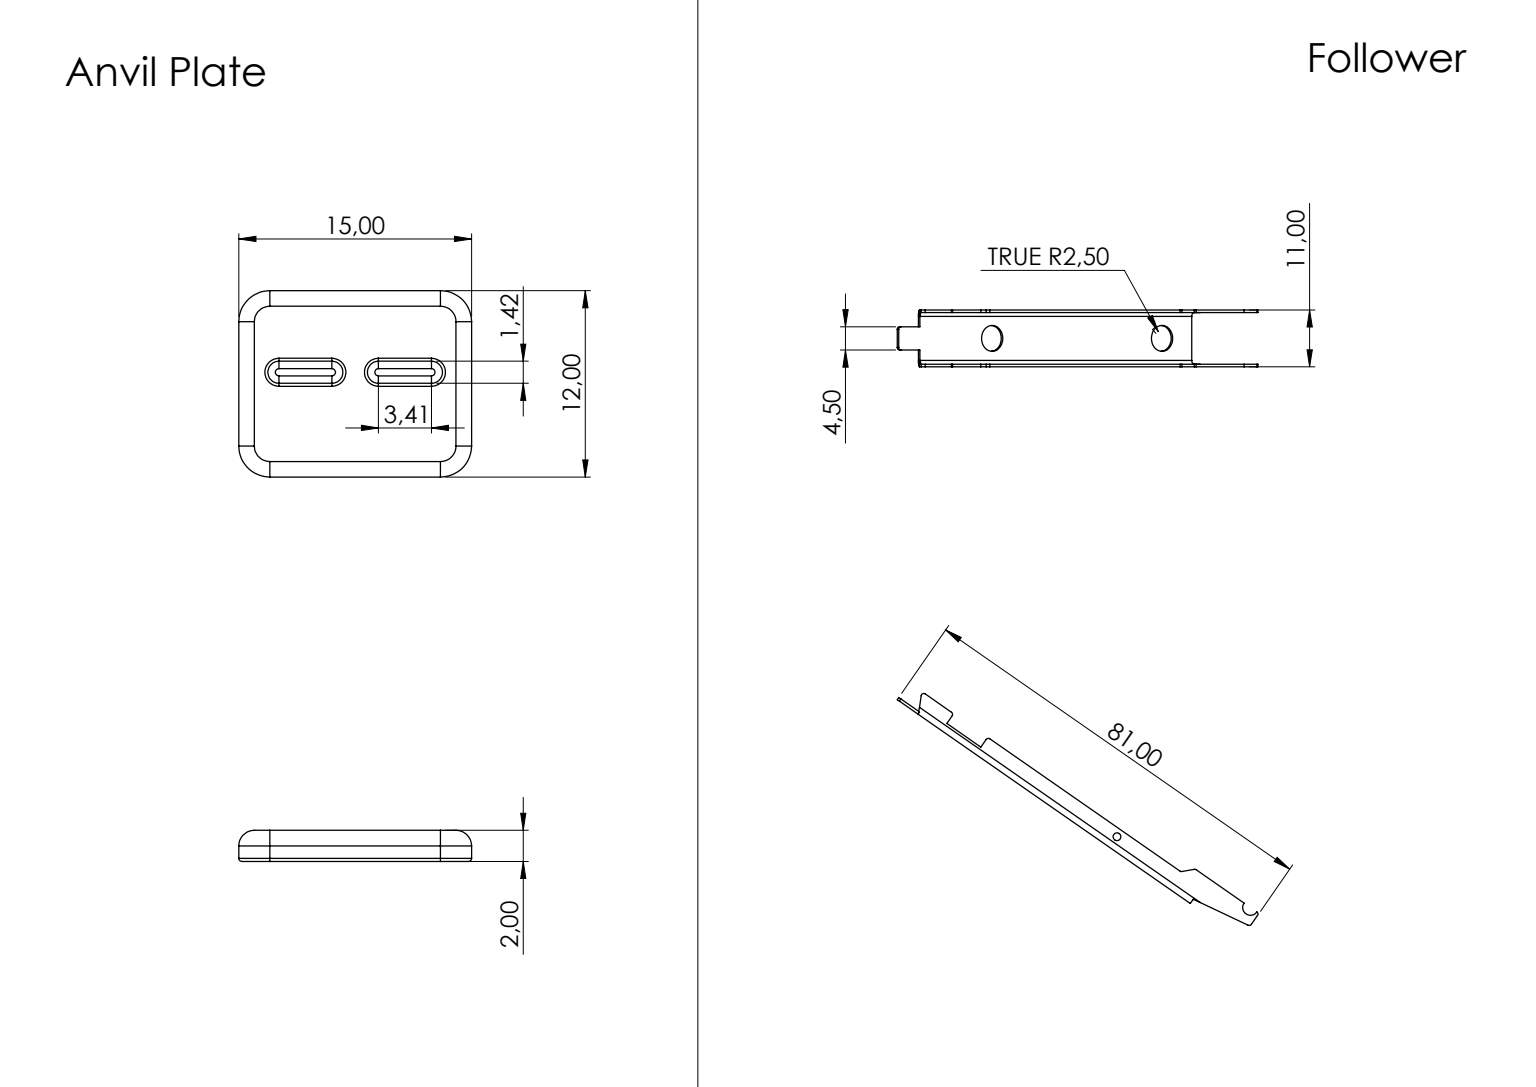
ISO-10303-21;
HEADER;
FILE_DESCRIPTION (('STEP AP214'),
    '1' );
FILE_NAME ('Anvil Plate.step',
    '2026-10-06T10:23:46',
    ( '' ),
    ( '' ),
    'SwSTEP 2.0',
    'SolidWorks 2020',
    '' );
FILE_SCHEMA (( 'AUTOMOTIVE_DESIGN' ));
ENDSEC;

DATA;
#13=EDGE_CURVE ( 'NONE', #2345, #1520, #288, .T. ) ;
#14=DIRECTION ( 'NONE',  ( 0.000000000000000000, 0.000000000000000000, 1.000000000000000000 ) ) ;
#20=CIRCLE ( 'NONE', #15263, 1.000000000000000888 ) ;
#27=CIRCLE ( 'NONE', #15267, 0.2000000000000057288 ) ;
#47=DIRECTION ( 'NONE',  ( 0.000000000000000000, 0.000000000000000000, -1.000000000000000000 ) ) ;
#57=DIRECTION ( 'NONE',  ( 0.000000000000000000, 1.000000000000000000, -3.469446951953613400E-15 ) ) ;
#77=ORIENTED_EDGE ( 'NONE', *, *, #24683, .F. ) ;
#92=ORIENTED_EDGE ( 'NONE', *, *, #24380, .T. ) ;
#97=EDGE_LOOP ( 'NONE', ( #25397, #5551, #19425, #6383 ) ) ;
#102=AXIS2_PLACEMENT_3D ( 'NONE', #15158, #5376, #18644 ) ;
#104=ADVANCED_FACE ( 'NONE', ( #4789 ), #24864, .T. ) ;
#145=CIRCLE ( 'NONE', #6320, 1.000000000000000888 ) ;
#158=AXIS2_PLACEMENT_3D ( 'NONE', #16213, #10429, #24064 ) ;
#165=LINE ( 'NONE', #13580, #21925 ) ;
#168=DIRECTION ( 'NONE',  ( 0.000000000000000000, 1.000000000000000000, -3.469446951953613400E-15 ) ) ;
#183=ORIENTED_EDGE ( 'NONE', *, *, #6628, .F. ) ;
#187=CARTESIAN_POINT ( 'NONE',  ( 43.23147868389327897, 41.90149715599300606, 79.87823623207322044 ) ) ;
#192=DIRECTION ( 'NONE',  ( 0.000000000000000000, 1.000000000000000000, -3.469446951953613400E-15 ) ) ;
#228=CARTESIAN_POINT ( 'NONE',  ( 32.81606138205700773, 36.92314894770294131, 81.17823623207323180 ) ) ;
#229=CYLINDRICAL_SURFACE ( 'NONE', #16961, 0.5000000000000004441 ) ;
#235=VERTEX_POINT ( 'NONE', #24984 ) ;
#237=DIRECTION ( 'NONE',  ( 1.000000000000000000, 0.000000000000000000, 0.000000000000000000 ) ) ;
#251=EDGE_CURVE ( 'NONE', #21293, #8440, #21528, .T. ) ;
#266=AXIS2_PLACEMENT_3D ( 'NONE', #24025, #20423, #700 ) ;
#288=CIRCLE ( 'NONE', #14300, 0.7106531558045068309 ) ;
#305=CARTESIAN_POINT ( 'NONE',  ( -3.469446951953610245E-16, 2.753545109730417678E-13, 79.37823623207336254 ) ) ;
#310=DIRECTION ( 'NONE',  ( 1.000000000000000000, 0.000000000000000000, 0.000000000000000000 ) ) ;
#329=CARTESIAN_POINT ( 'NONE',  ( 31.81606138205700418, 44.92314894770293421, 79.37823623207320622 ) ) ;
#346=EDGE_LOOP ( 'NONE', ( #3037, #6134, #10339, #6691 ) ) ;
#352=CARTESIAN_POINT ( 'NONE',  ( 33.40064408022072939, 41.90149715599300606, 79.37823623207322044 ) ) ;
#373=DIRECTION ( 'NONE',  ( -1.000000000000000000, -0.000000000000000000, -0.000000000000000000 ) ) ;
#407=DIRECTION ( 'NONE',  ( 1.734723475976805122E-16, 3.491481338843134933E-15, 1.000000000000000000 ) ) ;
#425=ADVANCED_FACE ( 'NONE', ( #18305 ), #23824, .T. ) ;
#460=CARTESIAN_POINT ( 'NONE',  ( 36.81465384343994884, 41.67000142393845152, 79.87823623207322044 ) ) ;
#485=TOROIDAL_SURFACE ( 'NONE', #1324, 1.000000000000000000, 1.000000000000000000 ) ;
#492=LINE ( 'NONE', #619, #7832 ) ;
#501=ORIENTED_EDGE ( 'NONE', *, *, #9098, .T. ) ;
#519=CARTESIAN_POINT ( 'NONE',  ( 31.01606138205699992, 44.92314894770294131, 81.17823623207320338 ) ) ;
#544=FACE_OUTER_BOUND ( 'NONE', #14731, .T. ) ;
#551=DIRECTION ( 'NONE',  ( 1.000000000000000000, 0.000000000000000000, 0.000000000000000000 ) ) ;
#565=DIRECTION ( 'NONE',  ( 0.000000000000000000, 0.000000000000000000, 1.000000000000000000 ) ) ;
#590=CARTESIAN_POINT ( 'NONE',  ( 33.40064408022072939, 42.38065457974295924, 79.52109337493035923 ) ) ;
#599=ORIENTED_EDGE ( 'NONE', *, *, #18942, .T. ) ;
#605=EDGE_LOOP ( 'NONE', ( #8949, #22189, #20198, #2594 ) ) ;
#613=CIRCLE ( 'NONE', #19551, 0.2314957320545540931 ) ;
#614=DIRECTION ( 'NONE',  ( 0.000000000000000000, 1.000000000000000000, -3.491481338843134933E-15 ) ) ;
#619=CARTESIAN_POINT ( 'NONE',  ( 43.23147868389327897, 40.76768529863396395, 79.37823623207322044 ) ) ;
#625=EDGE_CURVE ( 'NONE', #9404, #8440, #1536, .T. ) ;
#695=VECTOR ( 'NONE', #8729, 1000.000000000000000 ) ;
#700=DIRECTION ( 'NONE',  ( 0.000000000000000000, 0.000000000000000000, -1.000000000000000000 ) ) ;
#736=DIRECTION ( 'NONE',  ( 0.000000000000000000, 1.000000000000000000, 0.000000000000000000 ) ) ;
#757=DIRECTION ( 'NONE',  ( 0.000000000000000000, 0.000000000000000000, -1.000000000000000000 ) ) ;
#765=CIRCLE ( 'NONE', #17232, 0.5000000000000004441 ) ;
#774=CIRCLE ( 'NONE', #1188, 1.000000000000000888 ) ;
#778=EDGE_LOOP ( 'NONE', ( #24874, #9802, #12952, #15567 ) ) ;
#781=DIRECTION ( 'NONE',  ( 0.000000000000000000, -1.000000000000000000, 0.000000000000000000 ) ) ;
#784=AXIS2_PLACEMENT_3D ( 'NONE', #8790, #6837, #14690 ) ;
#810=ORIENTED_EDGE ( 'NONE', *, *, #4809, .T. ) ;
#822=ORIENTED_EDGE ( 'NONE', *, *, #5627, .F. ) ;
#840=CARTESIAN_POINT ( 'NONE',  ( 43.23147868389327897, 41.90149715599300606, 79.37823623207322044 ) ) ;
#849=CYLINDRICAL_SURFACE ( 'NONE', #21888, 1.000000000000000888 ) ;
#859=DIRECTION ( 'NONE',  ( 0.000000000000000000, -6.938893903907222067E-15, -1.000000000000000000 ) ) ;
#898=EDGE_CURVE ( 'NONE', #1130, #12932, #2769, .T. ) ;
#908=ORIENTED_EDGE ( 'NONE', *, *, #22325, .F. ) ;
#941=EDGE_LOOP ( 'NONE', ( #3944, #19997, #17589, #15115 ) ) ;
#947=VERTEX_POINT ( 'NONE', #19641 ) ;
#961=CARTESIAN_POINT ( 'NONE',  ( 43.81606138205700063, 36.92314894770294131, 81.17823623207323180 ) ) ;
#977=DIRECTION ( 'NONE',  ( 0.000000000000000000, 1.000000000000000000, 0.000000000000000000 ) ) ;
#1014=CARTESIAN_POINT ( 'NONE',  ( 31.81606138205700418, 44.92314894770294131, 80.37823623207322044 ) ) ;
#1056=CARTESIAN_POINT ( 'NONE',  ( 43.23147868389327897, 41.67000142393845152, 79.57823623207323749 ) ) ;
#1057=DIRECTION ( 'NONE',  ( 0.000000000000000000, -3.469446951953613400E-15, -1.000000000000000000 ) ) ;
#1085=VERTEX_POINT ( 'NONE', #2756 ) ;
#1122=CARTESIAN_POINT ( 'NONE',  ( 31.81606138205700418, 36.92314894770294131, 80.37823623207323465 ) ) ;
#1125=DIRECTION ( 'NONE',  ( 0.000000000000000000, 0.000000000000000000, -1.000000000000000000 ) ) ;
#1126=ORIENTED_EDGE ( 'NONE', *, *, #20228, .T. ) ;
#1130=VERTEX_POINT ( 'NONE', #12590 ) ;
#1132=ADVANCED_FACE ( 'NONE', ( #20048 ), #8586, .T. ) ;
#1138=ORIENTED_EDGE ( 'NONE', *, *, #21704, .T. ) ;
#1153=AXIS2_PLACEMENT_3D ( 'NONE', #1229, #14385, #6785 ) ;
#1188=AXIS2_PLACEMENT_3D ( 'NONE', #5142, #18661, #1125 ) ;
#1218=CARTESIAN_POINT ( 'NONE',  ( 33.40064408022072939, 42.57231754924293909, 79.37823623207320622 ) ) ;
#1229=CARTESIAN_POINT ( 'NONE',  ( 32.81606138205700773, 36.92314894770294131, 81.37823623207324886 ) ) ;
#1242=DIRECTION ( 'NONE',  ( 0.000000000000000000, 1.000000000000000000, 0.000000000000000000 ) ) ;
#1280=ORIENTED_EDGE ( 'NONE', *, *, #19495, .T. ) ;
#1323=DIRECTION ( 'NONE',  ( 0.000000000000000000, 0.000000000000000000, 1.000000000000000000 ) ) ;
#1324=AXIS2_PLACEMENT_3D ( 'NONE', #12607, #16567, #16067 ) ;
#1364=ORIENTED_EDGE ( 'NONE', *, *, #18759, .T. ) ;
#1385=EDGE_CURVE ( 'NONE', #23504, #12932, #9806, .T. ) ;
#1393=ORIENTED_EDGE ( 'NONE', *, *, #3030, .T. ) ;
#1416=CARTESIAN_POINT ( 'NONE',  ( 33.40064408022072939, 41.43850569188389699, 79.87823623207322044 ) ) ;
#1474=DIRECTION ( 'NONE',  ( 0.000000000000000000, 0.000000000000000000, -1.000000000000000000 ) ) ;
#1485=ORIENTED_EDGE ( 'NONE', *, *, #2006, .T. ) ;
#1493=DIRECTION ( 'NONE',  ( 1.000000000000000000, 0.000000000000000000, 0.000000000000000000 ) ) ;
#1498=CARTESIAN_POINT ( 'NONE',  ( 32.81606138205700773, 46.92314894770293421, 79.37823623207319201 ) ) ;
#1505=AXIS2_PLACEMENT_3D ( 'NONE', #21822, #6491, #10492 ) ;
#1508=CARTESIAN_POINT ( 'NONE',  ( 45.81606138205700063, 46.92314894770294131, 81.17823623207320338 ) ) ;
#1516=ORIENTED_EDGE ( 'NONE', *, *, #15444, .F. ) ;
#1520=VERTEX_POINT ( 'NONE', #21571 ) ;
#1536=CIRCLE ( 'NONE', #23353, 2.000000000000001776 ) ;
#1587=EDGE_LOOP ( 'NONE', ( #12351, #19325, #9251, #4956 ) ) ;
#1602=AXIS2_PLACEMENT_3D ( 'NONE', #22754, #16570, #1242 ) ;
#1605=EDGE_LOOP ( 'NONE', ( #92, #20381, #12875, #10899 ) ) ;
#1606=ORIENTED_EDGE ( 'NONE', *, *, #898, .F. ) ;
#1608=AXIS2_PLACEMENT_3D ( 'NONE', #10658, #22875, #18507 ) ;
#1612=VERTEX_POINT ( 'NONE', #19892 ) ;
#1669=ADVANCED_FACE ( 'NONE', ( #544 ), #17198, .T. ) ;
#1711=VERTEX_POINT ( 'NONE', #15887 ) ;
#1730=VECTOR ( 'NONE', #2169, 1000.000000000000000 ) ;
#1755=AXIS2_PLACEMENT_3D ( 'NONE', #3524, #11786, #21303 ) ;
#1772=ORIENTED_EDGE ( 'NONE', *, *, #6265, .T. ) ;
#1780=CARTESIAN_POINT ( 'NONE',  ( 36.81465384343994884, 41.67000142393845152, 79.57823623207323749 ) ) ;
#1819=CARTESIAN_POINT ( 'NONE',  ( 43.23147868389327897, 40.76768529863396395, 79.37823623207322044 ) ) ;
#1846=CIRCLE ( 'NONE', #16246, 0.5000000000000004441 ) ;
#1848=VERTEX_POINT ( 'NONE', #17046 ) ;
#1869=DIRECTION ( 'NONE',  ( -0.000000000000000000, -3.469446951953613400E-15, -1.000000000000000000 ) ) ;
#1875=CARTESIAN_POINT ( 'NONE',  ( 43.81606138205700063, 35.92314894770293421, 79.37823623207323465 ) ) ;
#1915=VERTEX_POINT ( 'NONE', #7122 ) ;
#1980=DIRECTION ( 'NONE',  ( 0.000000000000000000, -3.469446951953611033E-15, -1.000000000000000000 ) ) ;
#1984=TOROIDAL_SURFACE ( 'NONE', #17218, 1.000000000000000000, 1.000000000000000000 ) ;
#2000=AXIS2_PLACEMENT_3D ( 'NONE', #9286, #12766, #22537 ) ;
#2006=EDGE_CURVE ( 'NONE', #1520, #12430, #4412, .T. ) ;
#2033=ORIENTED_EDGE ( 'NONE', *, *, #9098, .F. ) ;
#2040=DIRECTION ( 'NONE',  ( 0.000000000000000000, 1.000000000000000000, -3.469446951953613400E-15 ) ) ;
#2042=DIRECTION ( 'NONE',  ( 0.000000000000000000, 3.469446951953613400E-15, 1.000000000000000000 ) ) ;
#2049=ORIENTED_EDGE ( 'NONE', *, *, #4239, .T. ) ;
#2067=DIRECTION ( 'NONE',  ( -0.000000000000000000, -3.469446951953613400E-15, -1.000000000000000000 ) ) ;
#2078=ADVANCED_FACE ( 'NONE', ( #15477 ), #9448, .T. ) ;
#2094=DIRECTION ( 'NONE',  ( 0.000000000000000000, 0.000000000000000000, -1.000000000000000000 ) ) ;
#2121=ORIENTED_EDGE ( 'NONE', *, *, #3983, .T. ) ;
#2142=VECTOR ( 'NONE', #25060, 1000.000000000000000 ) ;
#2154=EDGE_CURVE ( 'NONE', #3400, #23482, #8135, .T. ) ;
#2169=DIRECTION ( 'NONE',  ( -8.758115402030106693E-47, 1.000000000000000000, -3.469446951953613400E-15 ) ) ;
#2176=ORIENTED_EDGE ( 'NONE', *, *, #11481, .F. ) ;
#2182=AXIS2_PLACEMENT_3D ( 'NONE', #14350, #551, #47 ) ;
#2192=CARTESIAN_POINT ( 'NONE',  ( 33.40064408022072939, 42.57231754924293909, 79.37823623207320622 ) ) ;
#2201=AXIS2_PLACEMENT_3D ( 'NONE', #24335, #14817, #6707 ) ;
#2235=PRODUCT_DEFINITION_FORMATION_WITH_SPECIFIED_SOURCE ( 'ANY', '', #3964, .NOT_KNOWN. ) ;
#2249=EDGE_LOOP ( 'NONE', ( #3554, #6520, #9600, #21223 ) ) ;
#2279=CARTESIAN_POINT ( 'NONE',  ( 36.81465384343994884, 42.57231754924293909, 79.57823623207322328 ) ) ;
#2296=DIRECTION ( 'NONE',  ( 1.000000000000000000, -0.000000000000000000, -0.000000000000000000 ) ) ;
#2345=VERTEX_POINT ( 'NONE', #16392 ) ;
#2362=FACE_OUTER_BOUND ( 'NONE', #8970, .T. ) ;
#2364=FACE_OUTER_BOUND ( 'NONE', #2249, .T. ) ;
#2372=EDGE_CURVE ( 'NONE', #24574, #9515, #15507, .T. ) ;
#2380=DIRECTION ( 'NONE',  ( -8.758115402030106693E-47, 1.000000000000000000, -3.469446951953613400E-15 ) ) ;
#2454=CIRCLE ( 'NONE', #11126, 1.800000000000002931 ) ;
#2476=CARTESIAN_POINT ( 'NONE',  ( 32.81606138205700773, 45.92314894770293421, 79.37823623207320622 ) ) ;
#2480=ADVANCED_FACE ( 'NONE', ( #8934 ), #25385, .F. ) ;
#2497=LINE ( 'NONE', #6759, #16866 ) ;
#2528=FACE_OUTER_BOUND ( 'NONE', #778, .T. ) ;
#2533=CIRCLE ( 'NONE', #21472, 0.2000000000000057288 ) ;
#2553=AXIS2_PLACEMENT_3D ( 'NONE', #228, #14278, #21886 ) ;
#2594=ORIENTED_EDGE ( 'NONE', *, *, #5792, .F. ) ;
#2599=CIRCLE ( 'NONE', #7965, 0.2000000000000057288 ) ;
#2614=ADVANCED_FACE ( 'NONE', ( #12934 ), #22453, .F. ) ;
#2671=CARTESIAN_POINT ( 'NONE',  ( 32.81606138205700773, 36.92314894770293421, 79.37823623207323465 ) ) ;
#2691=DIRECTION ( 'NONE',  ( 0.000000000000000000, 0.000000000000000000, -1.000000000000000000 ) ) ;
#2725=DIRECTION ( 'NONE',  ( 0.000000000000000000, 1.000000000000000000, -3.469446951953613400E-15 ) ) ;
#2756=CARTESIAN_POINT ( 'NONE',  ( 30.81606138205700418, 44.92314894770294131, 80.37823623207322044 ) ) ;
#2757=VERTEX_POINT ( 'NONE', #15227 ) ;
#2763=ORIENTED_EDGE ( 'NONE', *, *, #11568, .F. ) ;
#2766=DIRECTION ( 'NONE',  ( 0.000000000000000000, 1.000000000000000000, -3.469446951953613400E-15 ) ) ;
#2769=LINE ( 'NONE', #16829, #695 ) ;
#2811=DIRECTION ( 'NONE',  ( 0.000000000000000000, 0.000000000000000000, 1.000000000000000000 ) ) ;
#2854=ORIENTED_EDGE ( 'NONE', *, *, #24360, .T. ) ;
#2907=ORIENTED_EDGE ( 'NONE', *, *, #20730, .T. ) ;
#2913=VECTOR ( 'NONE', #10280, 1000.000000000000000 ) ;
#2941=ORIENTED_EDGE ( 'NONE', *, *, #898, .T. ) ;
#2983=AXIS2_PLACEMENT_3D ( 'NONE', #20163, #8189, #565 ) ;
#3008=DIRECTION ( 'NONE',  ( 0.000000000000000000, 0.000000000000000000, 1.000000000000000000 ) ) ;
#3029=DIRECTION ( 'NONE',  ( 0.000000000000000000, -3.469446951953613400E-15, -1.000000000000000000 ) ) ;
#3030=EDGE_CURVE ( 'NONE', #7575, #19237, #18812, .T. ) ;
#3036=ORIENTED_EDGE ( 'NONE', *, *, #5474, .F. ) ;
#3037=ORIENTED_EDGE ( 'NONE', *, *, #7448, .F. ) ;
#3049=AXIS2_PLACEMENT_3D ( 'NONE', #8952, #9089, #8704 ) ;
#3069=UNCERTAINTY_MEASURE_WITH_UNIT (LENGTH_MEASURE( 1.000000000000000082E-05 ), #19515, 'distance_accuracy_value', 'NONE');
#3073=EDGE_CURVE ( 'NONE', #6274, #19237, #5359, .T. ) ;
#3285=DIRECTION ( 'NONE',  ( 0.000000000000000000, 1.000000000000000000, 0.000000000000000000 ) ) ;
#3301=DIRECTION ( 'NONE',  ( 0.000000000000000000, 1.000000000000000000, 0.000000000000000000 ) ) ;
#3315=DIRECTION ( 'NONE',  ( -0.000000000000000000, -3.469446951953613400E-15, -1.000000000000000000 ) ) ;
#3345=CIRCLE ( 'NONE', #19383, 0.5000000000000004441 ) ;
#3354=CARTESIAN_POINT ( 'NONE',  ( 39.81746892067405952, 42.57231754924293909, 79.37823623207320622 ) ) ;
#3387=VECTOR ( 'NONE', #13615, 1000.000000000000000 ) ;
#3394=CIRCLE ( 'NONE', #21099, 0.2000000000000057288 ) ;
#3400=VERTEX_POINT ( 'NONE', #5923 ) ;
#3404=( NAMED_UNIT ( * ) SI_UNIT ( $, .STERADIAN. ) SOLID_ANGLE_UNIT ( ) );
#3439=CARTESIAN_POINT ( 'NONE',  ( 36.81465384343994884, 40.76768529863396395, 79.37823623207322044 ) ) ;
#3473=PLANE ( 'NONE',  #18226 ) ;
#3482=ORIENTED_EDGE ( 'NONE', *, *, #13193, .T. ) ;
#3503=DIRECTION ( 'NONE',  ( -1.000000000000000000, 0.000000000000000000, 0.000000000000000000 ) ) ;
#3524=CARTESIAN_POINT ( 'NONE',  ( 39.81746892067405952, 42.57231754924293909, 79.57823623207322328 ) ) ;
#3534=DIRECTION ( 'NONE',  ( 0.000000000000000000, -1.000000000000000000, 0.000000000000000000 ) ) ;
#3537=( NAMED_UNIT ( * ) PLANE_ANGLE_UNIT ( ) SI_UNIT ( $, .RADIAN. ) );
#3554=ORIENTED_EDGE ( 'NONE', *, *, #13651, .T. ) ;
#3567=EDGE_CURVE ( 'NONE', #11430, #8412, #21363, .T. ) ;
#3569=AXIS2_PLACEMENT_3D ( 'NONE', #6497, #7937, #4190 ) ;
#3614=DIRECTION ( 'NONE',  ( 0.000000000000000000, 1.000000000000000000, 0.000000000000000000 ) ) ;
#3622=ORIENTED_EDGE ( 'NONE', *, *, #14918, .T. ) ;
#3690=ORIENTED_EDGE ( 'NONE', *, *, #17616, .T. ) ;
#3691=ORIENTED_EDGE ( 'NONE', *, *, #12095, .F. ) ;
#3692=CARTESIAN_POINT ( 'NONE',  ( 36.81465384343994884, 40.76768529863396395, 79.37823623207322044 ) ) ;
#3777=FILL_AREA_STYLE_COLOUR ( '', #11896 ) ;
#3785=VERTEX_POINT ( 'NONE', #10145 ) ;
#3800=CIRCLE ( 'NONE', #16984, 1.000000000000000888 ) ;
#3835=VERTEX_POINT ( 'NONE', #5541 ) ;
#3849=EDGE_LOOP ( 'NONE', ( #1772, #15717, #7269, #22855 ) ) ;
#3883=CIRCLE ( 'NONE', #18291, 1.000000000000000888 ) ;
#3890=DIRECTION ( 'NONE',  ( 0.000000000000000000, 0.000000000000000000, 1.000000000000000000 ) ) ;
#3896=LINE ( 'NONE', #23842, #15599 ) ;
#3922=ADVANCED_FACE ( 'NONE', ( #21372 ), #23415, .T. ) ;
#3944=ORIENTED_EDGE ( 'NONE', *, *, #16305, .T. ) ;
#3959=DIRECTION ( 'NONE',  ( 1.000000000000000000, 0.000000000000000000, 0.000000000000000000 ) ) ;
#3963=FACE_OUTER_BOUND ( 'NONE', #11280, .T. ) ;
#3964=PRODUCT ( 'Anvil Plate', 'Anvil Plate', '', ( #21040 ) ) ;
#3983=EDGE_CURVE ( 'NONE', #947, #1085, #19708, .T. ) ;
#4075=CARTESIAN_POINT ( 'NONE',  ( 39.81746892067405952, 41.67000142393845152, 79.57823623207323749 ) ) ;
#4097=FACE_OUTER_BOUND ( 'NONE', #18488, .T. ) ;
#4143=EDGE_CURVE ( 'NONE', #24976, #13846, #18108, .T. ) ;
#4190=DIRECTION ( 'NONE',  ( 0.000000000000000000, 1.000000000000000000, -3.469446951953613400E-15 ) ) ;
#4212=EDGE_LOOP ( 'NONE', ( #15416, #8055, #7794, #2176 ) ) ;
#4234=CIRCLE ( 'NONE', #14102, 1.000000000000000888 ) ;
#4239=EDGE_CURVE ( 'NONE', #9789, #15078, #2497, .T. ) ;
#4260=ORIENTED_EDGE ( 'NONE', *, *, #5474, .T. ) ;
#4277=CARTESIAN_POINT ( 'NONE',  ( 39.81746892067405952, 42.57231754924293909, 79.37823623207320622 ) ) ;
#4302=ORIENTED_EDGE ( 'NONE', *, *, #7371, .F. ) ;
#4355=CARTESIAN_POINT ( 'NONE',  ( 43.23147868389327897, 40.95934826813394380, 79.52109337493037344 ) ) ;
#4368=FACE_OUTER_BOUND ( 'NONE', #1587, .T. ) ;
#4412=CIRCLE ( 'NONE', #19209, 0.2000000000000057288 ) ;
#4450=CYLINDRICAL_SURFACE ( 'NONE', #5529, 0.2000000000000057288 ) ;
#4480=CARTESIAN_POINT ( 'NONE',  ( 39.81746892067405952, 40.76768529863396395, 79.37823623207322044 ) ) ;
#4496=FACE_OUTER_BOUND ( 'NONE', #6721, .T. ) ;
#4499=CARTESIAN_POINT ( 'NONE',  ( 45.61606138205700489, 44.92314894770294131, 81.17823623207320338 ) ) ;
#4527=LINE ( 'NONE', #18185, #7625 ) ;
#4539=VECTOR ( 'NONE', #14558, 1000.000000000000000 ) ;
#4566=EDGE_CURVE ( 'NONE', #1711, #21638, #19744, .T. ) ;
#4578=PLANE ( 'NONE',  #7457 ) ;
#4613=AXIS2_PLACEMENT_3D ( 'NONE', #5567, #2067, #9570 ) ;
#4672=DIRECTION ( 'NONE',  ( 0.000000000000000000, 0.000000000000000000, -1.000000000000000000 ) ) ;
#4693=CIRCLE ( 'NONE', #15330, 0.2000000000000057288 ) ;
#4699=ORIENTED_EDGE ( 'NONE', *, *, #4143, .F. ) ;
#4705=DIRECTION ( 'NONE',  ( -1.000000000000000000, 0.000000000000000000, 0.000000000000000000 ) ) ;
#4739=LINE ( 'NONE', #12612, #5832 ) ;
#4747=CARTESIAN_POINT ( 'NONE',  ( 45.81606138205700063, 34.92314894770293421, 79.37823623207323465 ) ) ;
#4762=DIRECTION ( 'NONE',  ( 1.000000000000000000, -0.000000000000000000, 0.000000000000000000 ) ) ;
#4787=CARTESIAN_POINT ( 'NONE',  ( 39.81746892067405952, 41.67000142393845152, 79.37823623207322044 ) ) ;
#4789=FACE_OUTER_BOUND ( 'NONE', #346, .T. ) ;
#4801=DIRECTION ( 'NONE',  ( 1.000000000000000000, 0.000000000000000000, -0.000000000000000000 ) ) ;
#4806=VECTOR ( 'NONE', #10198, 1000.000000000000000 ) ;
#4809=EDGE_CURVE ( 'NONE', #12932, #5707, #19729, .T. ) ;
#4879=EDGE_LOOP ( 'NONE', ( #20930, #20768, #17898, #4699 ) ) ;
#4882=CIRCLE ( 'NONE', #19283, 0.2314957320545540931 ) ;
#4932=VECTOR ( 'NONE', #17827, 1000.000000000000000 ) ;
#4956=ORIENTED_EDGE ( 'NONE', *, *, #18759, .F. ) ;
#4968=DIRECTION ( 'NONE',  ( 0.000000000000000000, 1.000000000000000000, -3.469446951953613400E-15 ) ) ;
#4974=CIRCLE ( 'NONE', #25113, 1.000000000000000888 ) ;
#4986=ADVANCED_FACE ( 'NONE', ( #14831 ), #20892, .F. ) ;
#4998=DIRECTION ( 'NONE',  ( 0.000000000000000000, 1.000000000000000000, 0.000000000000000000 ) ) ;
#5000=DIRECTION ( 'NONE',  ( 0.000000000000000000, -1.000000000000000000, 6.938893903907221278E-15 ) ) ;
#5026=CARTESIAN_POINT ( 'NONE',  ( 43.23147868389327897, 42.57231754924293909, 79.57823623207325170 ) ) ;
#5028=DIRECTION ( 'NONE',  ( -1.000000000000000000, 0.000000000000000000, 0.000000000000000000 ) ) ;
#5118=DIRECTION ( 'NONE',  ( 1.000000000000000000, 0.000000000000000000, 0.000000000000000000 ) ) ;
#5142=CARTESIAN_POINT ( 'NONE',  ( 43.81606138205700063, 35.92314894770294131, 80.37823623207323465 ) ) ;
#5143=VERTEX_POINT ( 'NONE', #7623 ) ;
#5146=EDGE_LOOP ( 'NONE', ( #23125, #7873, #11574, #23348 ) ) ;
#5175=ORIENTED_EDGE ( 'NONE', *, *, #5481, .F. ) ;
#5222=EDGE_LOOP ( 'NONE', ( #1126, #12846, #10725, #7105 ) ) ;
#5288=CIRCLE ( 'NONE', #1153, 1.800000000000002931 ) ;
#5359=CIRCLE ( 'NONE', #7767, 1.000000000000000888 ) ;
#5374=ORIENTED_EDGE ( 'NONE', *, *, #14624, .T. ) ;
#5376=DIRECTION ( 'NONE',  ( -0.000000000000000000, -3.469446951953613400E-15, -1.000000000000000000 ) ) ;
#5382=DIRECTION ( 'NONE',  ( 1.000000000000000000, -0.000000000000000000, -0.000000000000000000 ) ) ;
#5385=LINE ( 'NONE', #1498, #2142 ) ;
#5395=ORIENTED_EDGE ( 'NONE', *, *, #15441, .F. ) ;
#5424=EDGE_CURVE ( 'NONE', #13993, #1915, #14022, .T. ) ;
#5435=VECTOR ( 'NONE', #6960, 1000.000000000000000 ) ;
#5449=DIRECTION ( 'NONE',  ( -1.000000000000000000, 0.000000000000000000, 0.000000000000000000 ) ) ;
#5457=VECTOR ( 'NONE', #24680, 1000.000000000000000 ) ;
#5474=EDGE_CURVE ( 'NONE', #1520, #5143, #23469, .T. ) ;
#5481=EDGE_CURVE ( 'NONE', #19237, #8412, #20, .T. ) ;
#5482=FILL_AREA_STYLE ('',( #19256 ) ) ;
#5523=COLOUR_RGB ( '', 0.08235294, 0.09019608, 0.10196078) ;
#5529=AXIS2_PLACEMENT_3D ( 'NONE', #10249, #4705, #12317 ) ;
#5541=CARTESIAN_POINT ( 'NONE',  ( 32.81606138205700773, 46.92314894770294131, 81.17823623207318917 ) ) ;
#5551=ORIENTED_EDGE ( 'NONE', *, *, #24334, .F. ) ;
#5567=CARTESIAN_POINT ( 'NONE',  ( 43.81606138205700063, 44.92314894770294131, 81.17823623207320338 ) ) ;
#5570=CARTESIAN_POINT ( 'NONE',  ( 43.23147868389327897, 40.76768529863396395, 79.57823623207325170 ) ) ;
#5573=ADVANCED_FACE ( 'NONE', ( #15662 ), #17739, .T. ) ;
#5597=PRODUCT_DEFINITION_SHAPE ( 'NONE', 'NONE',  #23001 ) ;
#5599=EDGE_LOOP ( 'NONE', ( #1485, #22225, #16839, #23920 ) ) ;
#5627=EDGE_CURVE ( 'NONE', #6274, #24574, #17868, .T. ) ;
#5653=VECTOR ( 'NONE', #21399, 1000.000000000000000 ) ;
#5707=VERTEX_POINT ( 'NONE', #19918 ) ;
#5730=SHAPE_REPRESENTATION_RELATIONSHIP ( 'NONE' , 'NONE' ,  #10983, #9253 ) ;
#5792=EDGE_CURVE ( 'NONE', #1915, #16335, #8452, .T. ) ;
#5805=CARTESIAN_POINT ( 'NONE',  ( 33.40064408022072939, 40.95934826813394380, 79.52109337493035923 ) ) ;
#5821=DIRECTION ( 'NONE',  ( 0.000000000000000000, 1.000000000000000000, 0.000000000000000000 ) ) ;
#5832=VECTOR ( 'NONE', #20451, 1000.000000000000000 ) ;
#5865=LINE ( 'NONE', #20023, #9019 ) ;
#5890=ORIENTED_EDGE ( 'NONE', *, *, #5424, .T. ) ;
#5897=DIRECTION ( 'NONE',  ( 1.000000000000000000, -0.000000000000000000, 0.000000000000000000 ) ) ;
#5903=TOROIDAL_SURFACE ( 'NONE', #17027, 0.9023161253044896801, 0.2000000000000000111 ) ;
#5923=CARTESIAN_POINT ( 'NONE',  ( 43.23147868389327897, 42.57231754924293909, 79.37823623207320622 ) ) ;
#5965=CARTESIAN_POINT ( 'NONE',  ( 44.81606138205700063, 36.92314894770293421, 79.37823623207323465 ) ) ;
#5966=ADVANCED_FACE ( 'NONE', ( #15122 ), #12826, .T. ) ;
#5995=DIRECTION ( 'NONE',  ( 8.758115402030106693E-47, -1.000000000000000000, 3.469446951953613400E-15 ) ) ;
#6068=CARTESIAN_POINT ( 'NONE',  ( -3.469446951953610245E-16, 45.92314894770294131, 80.37823623207322044 ) ) ;
#6086=EDGE_CURVE ( 'NONE', #22567, #10123, #22398, .T. ) ;
#6134=ORIENTED_EDGE ( 'NONE', *, *, #9957, .F. ) ;
#6207=CIRCLE ( 'NONE', #21427, 1.000000000000000888 ) ;
#6242=DIRECTION ( 'NONE',  ( 1.000000000000000000, 0.000000000000000000, -0.000000000000000000 ) ) ;
#6248=FACE_BOUND ( 'NONE', #12703, .T. ) ;
#6250=EDGE_LOOP ( 'NONE', ( #15505, #9557, #24312, #22938 ) ) ;
#6261=VECTOR ( 'NONE', #20515, 1000.000000000000000 ) ;
#6263=AXIS2_PLACEMENT_3D ( 'NONE', #4787, #20508, #25073 ) ;
#6265=EDGE_CURVE ( 'NONE', #11430, #1915, #6362, .T. ) ;
#6266=LINE ( 'NONE', #24481, #6261 ) ;
#6272=EDGE_CURVE ( 'NONE', #22152, #17202, #3883, .T. ) ;
#6274=VERTEX_POINT ( 'NONE', #6731 ) ;
#6286=CIRCLE ( 'NONE', #7950, 0.2000000000000057288 ) ;
#6294=TOROIDAL_SURFACE ( 'NONE', #2553, 1.800000000000000044, 0.2000000000000000111 ) ;
#6315=CARTESIAN_POINT ( 'NONE',  ( 45.81606138205700063, 36.92314894770294131, 81.17823623207321759 ) ) ;
#6320=AXIS2_PLACEMENT_3D ( 'NONE', #1014, #20863, #12891 ) ;
#6336=CIRCLE ( 'NONE', #2201, 2.000000000000001776 ) ;
#6362=LINE ( 'NONE', #14335, #11719 ) ;
#6383=ORIENTED_EDGE ( 'NONE', *, *, #13, .F. ) ;
#6386=FACE_OUTER_BOUND ( 'NONE', #10307, .T. ) ;
#6419=DIRECTION ( 'NONE',  ( -1.000000000000000000, 0.000000000000000000, -0.000000000000000000 ) ) ;
#6467=CARTESIAN_POINT ( 'NONE',  ( 33.40064408022072939, 41.67000142393845152, 79.37823623207322044 ) ) ;
#6468=TOROIDAL_SURFACE ( 'NONE', #9357, 0.2314957320545545372, 0.5000000000000000000 ) ;
#6491=DIRECTION ( 'NONE',  ( 0.000000000000000000, 3.469446951953613400E-15, 1.000000000000000000 ) ) ;
#6497=CARTESIAN_POINT ( 'NONE',  ( 43.81606138205700063, 44.92314894770294131, 81.17823623207320338 ) ) ;
#6520=ORIENTED_EDGE ( 'NONE', *, *, #7973, .F. ) ;
#6531=CARTESIAN_POINT ( 'NONE',  ( 43.23147868389327897, 41.67000142393845152, 79.37823623207322044 ) ) ;
#6534=FACE_OUTER_BOUND ( 'NONE', #13113, .T. ) ;
#6562=AXIS2_PLACEMENT_3D ( 'NONE', #10788, #12984, #977 ) ;
#6602=DIRECTION ( 'NONE',  ( 0.000000000000000000, 1.000000000000000000, 0.000000000000000000 ) ) ;
#6603=DIRECTION ( 'NONE',  ( 1.734723475976805122E-16, 3.491481338843134933E-15, 1.000000000000000000 ) ) ;
#6628=EDGE_CURVE ( 'NONE', #13616, #5143, #613, .T. ) ;
#6678=ORIENTED_EDGE ( 'NONE', *, *, #3073, .F. ) ;
#6691=ORIENTED_EDGE ( 'NONE', *, *, #8106, .F. ) ;
#6707=DIRECTION ( 'NONE',  ( 0.000000000000000000, 1.000000000000000000, 0.000000000000000000 ) ) ;
#6721=EDGE_LOOP ( 'NONE', ( #11827, #21729, #21136, #13228 ) ) ;
#6731=CARTESIAN_POINT ( 'NONE',  ( 32.81606138205700773, 34.92314894770294131, 80.37823623207323465 ) ) ;
#6759=CARTESIAN_POINT ( 'NONE',  ( 0.000000000000000000, 35.12314894770293705, 81.37823623207324886 ) ) ;
#6785=DIRECTION ( 'NONE',  ( 0.000000000000000000, 1.000000000000000000, 0.000000000000000000 ) ) ;
#6786=EDGE_CURVE ( 'NONE', #13846, #10306, #15970, .T. ) ;
#6792=CARTESIAN_POINT ( 'NONE',  ( 32.81606138205700773, 44.92314894770294131, 81.37823623207322044 ) ) ;
#6798=FACE_OUTER_BOUND ( 'NONE', #11554, .T. ) ;
#6804=CARTESIAN_POINT ( 'NONE',  ( 32.81606138205700773, 35.12314894770294416, 81.37823623207324886 ) ) ;
#6833=CARTESIAN_POINT ( 'NONE',  ( 32.81606138205700773, 35.92314894770293421, 79.37823623207323465 ) ) ;
#6837=DIRECTION ( 'NONE',  ( 0.000000000000000000, 3.469446951953613400E-15, 1.000000000000000000 ) ) ;
#6867=EDGE_CURVE ( 'NONE', #1130, #19369, #1846, .T. ) ;
#6937=( GEOMETRIC_REPRESENTATION_CONTEXT ( 3 ) GLOBAL_UNCERTAINTY_ASSIGNED_CONTEXT ( ( #18240 ) ) GLOBAL_UNIT_ASSIGNED_CONTEXT ( ( #19502, #17076, #3404 ) ) REPRESENTATION_CONTEXT ( 'NONE', 'WORKASPACE' ) );
#6945=AXIS2_PLACEMENT_3D ( 'NONE', #24755, #5449, #1323 ) ;
#6947=DIRECTION ( 'NONE',  ( -0.000000000000000000, -3.469446951953613400E-15, -1.000000000000000000 ) ) ;
#6955=FACE_OUTER_BOUND ( 'NONE', #10604, .T. ) ;
#6960=DIRECTION ( 'NONE',  ( 8.758115402030106693E-47, -1.000000000000000000, 3.469446951953613400E-15 ) ) ;
#7000=DIRECTION ( 'NONE',  ( -8.758115402030106693E-47, 1.000000000000000000, -3.469446951953613400E-15 ) ) ;
#7022=CARTESIAN_POINT ( 'NONE',  ( 33.40064408022072939, 41.43850569188389699, 79.37823623207322044 ) ) ;
#7038=CARTESIAN_POINT ( 'NONE',  ( 39.81746892067405952, 42.38065457974295924, 79.52109337493037344 ) ) ;
#7058=CARTESIAN_POINT ( 'NONE',  ( 43.81606138205700063, 36.92314894770293421, 79.37823623207323465 ) ) ;
#7074=DIRECTION ( 'NONE',  ( 0.000000000000000000, 1.000000000000000000, 0.000000000000000000 ) ) ;
#7105=ORIENTED_EDGE ( 'NONE', *, *, #23720, .T. ) ;
#7111=ORIENTED_EDGE ( 'NONE', *, *, #16308, .T. ) ;
#7122=CARTESIAN_POINT ( 'NONE',  ( 30.81606138205700418, 36.92314894770294131, 81.17823623207323180 ) ) ;
#7143=FACE_OUTER_BOUND ( 'NONE', #23302, .T. ) ;
#7174=FACE_OUTER_BOUND ( 'NONE', #15055, .T. ) ;
#7269=ORIENTED_EDGE ( 'NONE', *, *, #14948, .T. ) ;
#7295=ORIENTED_EDGE ( 'NONE', *, *, #11580, .T. ) ;
#7339=EDGE_LOOP ( 'NONE', ( #24898, #24455, #14377, #24400 ) ) ;
#7344=AXIS2_PLACEMENT_3D ( 'NONE', #21061, #7533, #21188 ) ;
#7365=CARTESIAN_POINT ( 'NONE',  ( 43.81606138205700063, 46.92314894770293421, 79.37823623207319201 ) ) ;
#7371=EDGE_CURVE ( 'NONE', #1612, #13993, #20713, .T. ) ;
#7448=EDGE_CURVE ( 'NONE', #24976, #19369, #3394, .T. ) ;
#7451=ORIENTED_EDGE ( 'NONE', *, *, #11713, .F. ) ;
#7457=AXIS2_PLACEMENT_3D ( 'NONE', #305, #20289, #57 ) ;
#7494=AXIS2_PLACEMENT_3D ( 'NONE', #6792, #24671, #3301 ) ;
#7501=ORIENTED_EDGE ( 'NONE', *, *, #6272, .T. ) ;
#7504=SHAPE_DEFINITION_REPRESENTATION ( #5597, #10983 ) ;
#7530=DIRECTION ( 'NONE',  ( 1.000000000000000000, 0.000000000000000000, 0.000000000000000000 ) ) ;
#7533=DIRECTION ( 'NONE',  ( 1.000000000000000000, 0.000000000000000000, 0.000000000000000000 ) ) ;
#7575=VERTEX_POINT ( 'NONE', #1875 ) ;
#7592=AXIS2_PLACEMENT_3D ( 'NONE', #9094, #9224, #3008 ) ;
#7623=CARTESIAN_POINT ( 'NONE',  ( 43.23147868389327897, 41.43850569188389699, 79.87823623207322044 ) ) ;
#7625=VECTOR ( 'NONE', #8653, 1000.000000000000000 ) ;
#7670=SURFACE_STYLE_FILL_AREA ( #5482 ) ;
#7717=LINE ( 'NONE', #9909, #12848 ) ;
#7737=ORIENTED_EDGE ( 'NONE', *, *, #20228, .F. ) ;
#7743=EDGE_CURVE ( 'NONE', #2757, #13616, #6266, .T. ) ;
#7767=AXIS2_PLACEMENT_3D ( 'NONE', #9168, #10959, #22549 ) ;
#7794=ORIENTED_EDGE ( 'NONE', *, *, #16305, .F. ) ;
#7798=SURFACE_STYLE_USAGE ( .BOTH. , #9484 ) ;
#7832=VECTOR ( 'NONE', #237, 1000.000000000000000 ) ;
#7873=ORIENTED_EDGE ( 'NONE', *, *, #5424, .F. ) ;
#7895=EDGE_CURVE ( 'NONE', #1085, #11430, #15473, .T. ) ;
#7927=CIRCLE ( 'NONE', #7494, 1.800000000000002931 ) ;
#7937=DIRECTION ( 'NONE',  ( -0.000000000000000000, -3.469446951953613400E-15, -1.000000000000000000 ) ) ;
#7943=AXIS2_PLACEMENT_3D ( 'NONE', #460, #23907, #22237 ) ;
#7950=AXIS2_PLACEMENT_3D ( 'NONE', #8453, #23894, #19920 ) ;
#7952=EDGE_LOOP ( 'NONE', ( #13257, #15522, #18354, #1606 ) ) ;
#7965=AXIS2_PLACEMENT_3D ( 'NONE', #14476, #16524, #12567 ) ;
#7968=CARTESIAN_POINT ( 'NONE',  ( 36.81465384343994884, 40.95934826813394380, 79.52109337493037344 ) ) ;
#7973=EDGE_CURVE ( 'NONE', #9136, #3785, #2454, .T. ) ;
#8012=ORIENTED_EDGE ( 'NONE', *, *, #24661, .T. ) ;
#8049=ORIENTED_EDGE ( 'NONE', *, *, #17211, .T. ) ;
#8055=ORIENTED_EDGE ( 'NONE', *, *, #19946, .F. ) ;
#8065=FACE_OUTER_BOUND ( 'NONE', #23914, .T. ) ;
#8075=ORIENTED_EDGE ( 'NONE', *, *, #4143, .T. ) ;
#8082=ORIENTED_EDGE ( 'NONE', *, *, #21225, .T. ) ;
#8094=DIRECTION ( 'NONE',  ( 0.000000000000000000, 1.000000000000000000, 0.000000000000000000 ) ) ;
#8106=EDGE_CURVE ( 'NONE', #19369, #23504, #10194, .T. ) ;
#8135=LINE ( 'NONE', #4277, #4806 ) ;
#8177=AXIS2_PLACEMENT_3D ( 'NONE', #12636, #15761, #21567 ) ;
#8189=DIRECTION ( 'NONE',  ( -1.000000000000000000, 0.000000000000000000, 0.000000000000000000 ) ) ;
#8210=DIRECTION ( 'NONE',  ( -8.758115402030106693E-47, 1.000000000000000000, -3.469446951953613400E-15 ) ) ;
#8220=ORIENTED_EDGE ( 'NONE', *, *, #12827, .T. ) ;
#8246=CARTESIAN_POINT ( 'NONE',  ( 45.81606138205700063, 44.92314894770294131, 81.17823623207320338 ) ) ;
#8250=CIRCLE ( 'NONE', #9925, 0.9023161253044892360 ) ;
#8270=DIRECTION ( 'NONE',  ( -0.000000000000000000, -3.469446951953613400E-15, -1.000000000000000000 ) ) ;
#8308=DIRECTION ( 'NONE',  ( 0.000000000000000000, 0.000000000000000000, -1.000000000000000000 ) ) ;
#8350=LINE ( 'NONE', #4355, #2913 ) ;
#8412=VERTEX_POINT ( 'NONE', #17386 ) ;
#8440=VERTEX_POINT ( 'NONE', #11732 ) ;
#8452=LINE ( 'NONE', #20168, #20595 ) ;
#8453=CARTESIAN_POINT ( 'NONE',  ( 43.81606138205700063, 35.12314894770293705, 81.17823623207323180 ) ) ;
#8475=CARTESIAN_POINT ( 'NONE',  ( 33.40064408022072939, 40.76768529863396395, 79.37823623207322044 ) ) ;
#8483=DIRECTION ( 'NONE',  ( -0.000000000000000000, -3.469446951953613400E-15, -1.000000000000000000 ) ) ;
#8516=DIRECTION ( 'NONE',  ( 0.000000000000000000, 1.000000000000000000, -3.469446951953613400E-15 ) ) ;
#8561=DIRECTION ( 'NONE',  ( 0.000000000000000000, 0.000000000000000000, 1.000000000000000000 ) ) ;
#8586=CYLINDRICAL_SURFACE ( 'NONE', #266, 0.2000000000000057288 ) ;
#8635=AXIS2_PLACEMENT_3D ( 'NONE', #14455, #17955, #781 ) ;
#8653=DIRECTION ( 'NONE',  ( 1.000000000000000000, 0.000000000000000000, 0.000000000000000000 ) ) ;
#8704=DIRECTION ( 'NONE',  ( 1.734723475976805122E-16, 0.000000000000000000, 1.000000000000000000 ) ) ;
#8729=DIRECTION ( 'NONE',  ( -1.000000000000000000, 0.000000000000000000, 0.000000000000000000 ) ) ;
#8734=DIRECTION ( 'NONE',  ( 0.000000000000000000, 1.000000000000000000, -3.469446951953613400E-15 ) ) ;
#8740=DIRECTION ( 'NONE',  ( 0.000000000000000000, 3.469446951953611033E-15, 1.000000000000000000 ) ) ;
#8782=DIRECTION ( 'NONE',  ( -1.000000000000000000, 0.000000000000000000, 0.000000000000000000 ) ) ;
#8785=CIRCLE ( 'NONE', #21120, 0.2000000000000057288 ) ;
#8790=CARTESIAN_POINT ( 'NONE',  ( 33.40064408022072939, 41.67000142393845152, 79.37823623207322044 ) ) ;
#8819=DIRECTION ( 'NONE',  ( 0.000000000000000000, 0.000000000000000000, -1.000000000000000000 ) ) ;
#8934=FACE_OUTER_BOUND ( 'NONE', #11469, .T. ) ;
#8949=ORIENTED_EDGE ( 'NONE', *, *, #10543, .F. ) ;
#8952=CARTESIAN_POINT ( 'NONE',  ( 45.81606138205700063, 46.92314894770293421, 79.37823623207319201 ) ) ;
#8970=EDGE_LOOP ( 'NONE', ( #7111, #17634, #22349, #9503 ) ) ;
#8971=CARTESIAN_POINT ( 'NONE',  ( 31.01606138205700347, 44.92314894770294131, 81.37823623207322044 ) ) ;
#9019=VECTOR ( 'NONE', #13724, 1000.000000000000000 ) ;
#9026=CARTESIAN_POINT ( 'NONE',  ( 36.81465384343994884, 41.43850569188389699, 79.37823623207322044 ) ) ;
#9049=ORIENTED_EDGE ( 'NONE', *, *, #16308, .F. ) ;
#9061=DIRECTION ( 'NONE',  ( 1.000000000000000000, 0.000000000000000000, -0.000000000000000000 ) ) ;
#9078=CYLINDRICAL_SURFACE ( 'NONE', #25208, 0.2000000000000057288 ) ;
#9089=DIRECTION ( 'NONE',  ( -1.000000000000000000, 6.018531076210103283E-31, 1.734723475976805122E-16 ) ) ;
#9094=CARTESIAN_POINT ( 'NONE',  ( 43.23147868389327897, 40.76768529863396395, 79.57823623207323749 ) ) ;
#9098=EDGE_CURVE ( 'NONE', #24470, #2345, #4527, .T. ) ;
#9125=VERTEX_POINT ( 'NONE', #16482 ) ;
#9136=VERTEX_POINT ( 'NONE', #20234 ) ;
#9163=DIRECTION ( 'NONE',  ( -0.000000000000000000, -3.469446951953613400E-15, -1.000000000000000000 ) ) ;
#9168=CARTESIAN_POINT ( 'NONE',  ( 32.81606138205700773, 35.92314894770294131, 80.37823623207323465 ) ) ;
#9170=DIRECTION ( 'NONE',  ( 1.734723475976805122E-16, 3.491481338843134933E-15, 1.000000000000000000 ) ) ;
#9186=CARTESIAN_POINT ( 'NONE',  ( 30.81606138205700418, 46.92314894770293421, 79.37823623207319201 ) ) ;
#9224=DIRECTION ( 'NONE',  ( -1.000000000000000000, 0.000000000000000000, 0.000000000000000000 ) ) ;
#9251=ORIENTED_EDGE ( 'NONE', *, *, #9367, .F. ) ;
#9253=ADVANCED_BREP_SHAPE_REPRESENTATION ( '', ( #25350, #2000 ), #16613 ) ;
#9286=CARTESIAN_POINT ( 'NONE',  ( 0.000000000000000000, 0.000000000000000000, 0.000000000000000000 ) ) ;
#9357=AXIS2_PLACEMENT_3D ( 'NONE', #6467, #18446, #16756 ) ;
#9367=EDGE_CURVE ( 'NONE', #235, #12986, #13280, .T. ) ;
#9388=AXIS2_PLACEMENT_3D ( 'NONE', #16011, #17967, #168 ) ;
#9404=VERTEX_POINT ( 'NONE', #22801 ) ;
#9448=PLANE ( 'NONE',  #17158 ) ;
#9484=SURFACE_SIDE_STYLE ('',( #7670 ) ) ;
#9503=ORIENTED_EDGE ( 'NONE', *, *, #7895, .F. ) ;
#9515=VERTEX_POINT ( 'NONE', #21503 ) ;
#9519=CARTESIAN_POINT ( 'NONE',  ( 43.81606138205700063, 45.92314894770293421, 79.37823623207320622 ) ) ;
#9552=ADVANCED_FACE ( 'NONE', ( #13779 ), #3473, .F. ) ;
#9557=ORIENTED_EDGE ( 'NONE', *, *, #14726, .F. ) ;
#9570=DIRECTION ( 'NONE',  ( 0.000000000000000000, 1.000000000000000000, 0.000000000000000000 ) ) ;
#9598=ADVANCED_FACE ( 'NONE', ( #18155 ), #6294, .T. ) ;
#9600=ORIENTED_EDGE ( 'NONE', *, *, #13243, .F. ) ;
#9604=CIRCLE ( 'NONE', #158, 0.2000000000000057288 ) ;
#9670=ORIENTED_EDGE ( 'NONE', *, *, #3073, .T. ) ;
#9678=DIRECTION ( 'NONE',  ( 0.000000000000000000, 0.000000000000000000, 1.000000000000000000 ) ) ;
#9712=ORIENTED_EDGE ( 'NONE', *, *, #20420, .F. ) ;
#9729=CARTESIAN_POINT ( 'NONE',  ( 31.01606138205699992, 36.92314894770294131, 81.17823623207323180 ) ) ;
#9789=VERTEX_POINT ( 'NONE', #6804 ) ;
#9802=ORIENTED_EDGE ( 'NONE', *, *, #20730, .F. ) ;
#9806=CIRCLE ( 'NONE', #22534, 0.5000000000000004441 ) ;
#9820=DIRECTION ( 'NONE',  ( 8.758115402030106693E-47, -1.000000000000000000, 3.469446951953613400E-15 ) ) ;
#9857=EDGE_CURVE ( 'NONE', #21638, #7575, #4234, .T. ) ;
#9866=CARTESIAN_POINT ( 'NONE',  ( 43.81606138205700063, 46.92314894770294131, 81.17823623207318917 ) ) ;
#9880=ORIENTED_EDGE ( 'NONE', *, *, #14297, .T. ) ;
#9908=EDGE_LOOP ( 'NONE', ( #9880, #15629, #23440, #15210 ) ) ;
#9909=CARTESIAN_POINT ( 'NONE',  ( 45.81606138205700063, 44.92314894770293421, 79.37823623207320622 ) ) ;
#9925=AXIS2_PLACEMENT_3D ( 'NONE', #6531, #14390, #8094 ) ;
#9957=EDGE_CURVE ( 'NONE', #17769, #24976, #23523, .T. ) ;
#9995=FACE_OUTER_BOUND ( 'NONE', #19170, .T. ) ;
#10007=CARTESIAN_POINT ( 'NONE',  ( 30.81606138205700418, 44.92314894770293421, 79.37823623207320622 ) ) ;
#10032=ORIENTED_EDGE ( 'NONE', *, *, #3567, .T. ) ;
#10110=VERTEX_POINT ( 'NONE', #10267 ) ;
#10120=ORIENTED_EDGE ( 'NONE', *, *, #25442, .F. ) ;
#10123=VERTEX_POINT ( 'NONE', #13876 ) ;
#10145=CARTESIAN_POINT ( 'NONE',  ( 43.81606138205700063, 46.72314894770294558, 81.37823623207320622 ) ) ;
#10194=LINE ( 'NONE', #24327, #4539 ) ;
#10198=DIRECTION ( 'NONE',  ( -1.000000000000000000, 0.000000000000000000, 0.000000000000000000 ) ) ;
#10211=LINE ( 'NONE', #23972, #11839 ) ;
#10222=CYLINDRICAL_SURFACE ( 'NONE', #15768, 2.000000000000001776 ) ;
#10249=CARTESIAN_POINT ( 'NONE',  ( 45.81606138205700063, 35.12314894770293705, 81.17823623207323180 ) ) ;
#10256=FACE_OUTER_BOUND ( 'NONE', #10786, .T. ) ;
#10267=CARTESIAN_POINT ( 'NONE',  ( 39.81746892067405952, 41.43850569188389699, 79.87823623207322044 ) ) ;
#10270=CARTESIAN_POINT ( 'NONE',  ( 31.01606138205699992, 36.92314894770294131, 81.37823623207324886 ) ) ;
#10271=AXIS2_PLACEMENT_3D ( 'NONE', #1122, #5000, #859 ) ;
#10280=DIRECTION ( 'NONE',  ( -1.000000000000000000, 0.000000000000000000, 0.000000000000000000 ) ) ;
#10282=VERTEX_POINT ( 'NONE', #8971 ) ;
#10302=ORIENTED_EDGE ( 'NONE', *, *, #3983, .F. ) ;
#10306=VERTEX_POINT ( 'NONE', #1218 ) ;
#10307=EDGE_LOOP ( 'NONE', ( #8049, #4302, #18356, #18215 ) ) ;
#10339=ORIENTED_EDGE ( 'NONE', *, *, #13272, .F. ) ;
#10357=CYLINDRICAL_SURFACE ( 'NONE', #2182, 0.2000000000000057288 ) ;
#10388=TOROIDAL_SURFACE ( 'NONE', #11624, 0.9023161253044896801, 0.2000000000000000111 ) ;
#10398=LINE ( 'NONE', #329, #20293 ) ;
#10421=ADVANCED_FACE ( 'NONE', ( #20556 ), #23559, .T. ) ;
#10429=DIRECTION ( 'NONE',  ( -1.000000000000000000, 0.000000000000000000, 0.000000000000000000 ) ) ;
#10452=DIRECTION ( 'NONE',  ( -0.000000000000000000, -3.469446951953613400E-15, -1.000000000000000000 ) ) ;
#10457=VECTOR ( 'NONE', #9170, 1000.000000000000000 ) ;
#10483=LINE ( 'NONE', #14462, #12072 ) ;
#10492=DIRECTION ( 'NONE',  ( 0.000000000000000000, 1.000000000000000000, 0.000000000000000000 ) ) ;
#10543=EDGE_CURVE ( 'NONE', #11605, #1915, #14144, .T. ) ;
#10548=DIRECTION ( 'NONE',  ( 0.000000000000000000, 0.000000000000000000, -1.000000000000000000 ) ) ;
#10561=ORIENTED_EDGE ( 'NONE', *, *, #15581, .F. ) ;
#10593=AXIS2_PLACEMENT_3D ( 'NONE', #16520, #1057, #16658 ) ;
#10604=EDGE_LOOP ( 'NONE', ( #9670, #21631, #908, #822 ) ) ;
#10606=CARTESIAN_POINT ( 'NONE',  ( 32.81606138205700773, 44.92314894770293421, 79.37823623207320622 ) ) ;
#10658=CARTESIAN_POINT ( 'NONE',  ( 33.40064408022072939, 41.67000142393845152, 79.87823623207322044 ) ) ;
#10706=CARTESIAN_POINT ( 'NONE',  ( 43.81606138205700063, 45.92314894770293421, 80.37823623207322044 ) ) ;
#10710=FACE_OUTER_BOUND ( 'NONE', #1605, .T. ) ;
#10725=ORIENTED_EDGE ( 'NONE', *, *, #6628, .T. ) ;
#10727=ORIENTED_EDGE ( 'NONE', *, *, #13193, .F. ) ;
#10757=ADVANCED_FACE ( 'NONE', ( #24613 ), #5903, .T. ) ;
#10786=EDGE_LOOP ( 'NONE', ( #15532, #8220, #22506, #25370 ) ) ;
#10788=CARTESIAN_POINT ( 'NONE',  ( 36.81465384343994884, 41.67000142393845152, 79.37823623207322044 ) ) ;
#10870=ORIENTED_EDGE ( 'NONE', *, *, #11241, .F. ) ;
#10884=PLANE ( 'NONE',  #3049 ) ;
#10899=ORIENTED_EDGE ( 'NONE', *, *, #9857, .F. ) ;
#10959=DIRECTION ( 'NONE',  ( 1.000000000000000000, 0.000000000000000000, 0.000000000000000000 ) ) ;
#10983=SHAPE_REPRESENTATION ( 'Anvil Plate', ( #2000 ), #16613 ) ;
#11036=AXIS2_PLACEMENT_3D ( 'NONE', #16857, #8270, #13125 ) ;
#11051=ORIENTED_EDGE ( 'NONE', *, *, #12598, .T. ) ;
#11055=ADVANCED_FACE ( 'NONE', ( #13653 ), #15792, .F. ) ;
#11101=ADVANCED_FACE ( 'NONE', ( #4368 ), #229, .F. ) ;
#11107=DIRECTION ( 'NONE',  ( 1.000000000000000000, -6.018531076210103283E-31, -1.734723475976805122E-16 ) ) ;
#11126=AXIS2_PLACEMENT_3D ( 'NONE', #21404, #15857, #5821 ) ;
#11155=ADVANCED_FACE ( 'NONE', ( #4496 ), #15952, .F. ) ;
#11220=AXIS2_PLACEMENT_3D ( 'NONE', #2279, #6419, #18385 ) ;
#11223=AXIS2_PLACEMENT_3D ( 'NONE', #13149, #5028, #16746 ) ;
#11232=CIRCLE ( 'NONE', #15743, 2.000000000000001776 ) ;
#11241=EDGE_CURVE ( 'NONE', #9515, #9404, #22394, .T. ) ;
#11280=EDGE_LOOP ( 'NONE', ( #11783, #24766, #4260, #183 ) ) ;
#11282=CIRCLE ( 'NONE', #14955, 1.000000000000000888 ) ;
#11298=PRESENTATION_STYLE_ASSIGNMENT (( #7798 ) ) ;
#11413=( LENGTH_UNIT ( ) NAMED_UNIT ( * ) SI_UNIT ( .MILLI., .METRE. ) );
#11424=CLOSED_SHELL ( 'NONE', ( #4986, #22630, #13704, #11155, #24727, #9552, #18224, #15165, #15608, #17115, #17498, #425, #23172, #19469, #17813, #14745, #16321, #17628, #22832, #2078, #11101, #11055, #21857, #2614, #13633, #2480, #19481, #24415, #104, #17772, #3922, #20278, #12739, #10757, #5573, #5966, #12318, #1669, #9598, #12264, #13606, #21360, #10421, #1132 ) ) ;
#11430=VERTEX_POINT ( 'NONE', #14655 ) ;
#11448=VECTOR ( 'NONE', #24150, 1000.000000000000000 ) ;
#11469=EDGE_LOOP ( 'NONE', ( #22198, #18960, #10727, #7737 ) ) ;
#11472=DIRECTION ( 'NONE',  ( 0.000000000000000000, -3.469446951953613400E-15, -1.000000000000000000 ) ) ;
#11481=EDGE_CURVE ( 'NONE', #17202, #1848, #17500, .T. ) ;
#11506=DIRECTION ( 'NONE',  ( 0.000000000000000000, 1.000000000000000000, -3.469446951953613400E-15 ) ) ;
#11554=EDGE_LOOP ( 'NONE', ( #8012, #10870, #12642, #23769 ) ) ;
#11555=CARTESIAN_POINT ( 'NONE',  ( 44.81606138205700063, 44.92314894770293421, 80.37823623207322044 ) ) ;
#11568=EDGE_CURVE ( 'NONE', #17202, #947, #3800, .T. ) ;
#11570=AXIS2_PLACEMENT_3D ( 'NONE', #4075, #1869, #192 ) ;
#11574=ORIENTED_EDGE ( 'NONE', *, *, #17211, .F. ) ;
#11580=EDGE_CURVE ( 'NONE', #947, #3835, #5385, .T. ) ;
#11602=CARTESIAN_POINT ( 'NONE',  ( 36.81465384343994884, 42.38065457974295924, 79.52109337493035923 ) ) ;
#11605=VERTEX_POINT ( 'NONE', #10270 ) ;
#11624=AXIS2_PLACEMENT_3D ( 'NONE', #24290, #18273, #8734 ) ;
#11646=EDGE_CURVE ( 'NONE', #8412, #22152, #10398, .T. ) ;
#11694=VERTEX_POINT ( 'NONE', #590 ) ;
#11713=EDGE_CURVE ( 'NONE', #235, #1130, #12887, .T. ) ;
#11719=VECTOR ( 'NONE', #407, 1000.000000000000000 ) ;
#11732=CARTESIAN_POINT ( 'NONE',  ( 43.81606138205700063, 46.92314894770294131, 80.37823623207322044 ) ) ;
#11783=ORIENTED_EDGE ( 'NONE', *, *, #15398, .F. ) ;
#11786=DIRECTION ( 'NONE',  ( -1.000000000000000000, 0.000000000000000000, -0.000000000000000000 ) ) ;
#11799=CARTESIAN_POINT ( 'NONE',  ( 32.81606138205700773, 44.92314894770294131, 81.17823623207320338 ) ) ;
#11809=ORIENTED_EDGE ( 'NONE', *, *, #19821, .F. ) ;
#11816=DIRECTION ( 'NONE',  ( 1.000000000000000000, -0.000000000000000000, -0.000000000000000000 ) ) ;
#11827=ORIENTED_EDGE ( 'NONE', *, *, #12974, .T. ) ;
#11839=VECTOR ( 'NONE', #19606, 1000.000000000000000 ) ;
#11842=ORIENTED_EDGE ( 'NONE', *, *, #9957, .T. ) ;
#11861=CARTESIAN_POINT ( 'NONE',  ( 36.81465384343994884, 41.67000142393845152, 79.37823623207322044 ) ) ;
#11896=COLOUR_RGB ( '', 0.08235294, 0.09019608, 0.10196078) ;
#11958=ORIENTED_EDGE ( 'NONE', *, *, #18218, .T. ) ;
#11994=CARTESIAN_POINT ( 'NONE',  ( 39.81746892067405952, 41.90149715599300606, 79.37823623207322044 ) ) ;
#12072=VECTOR ( 'NONE', #22318, 1000.000000000000000 ) ;
#12095=EDGE_CURVE ( 'NONE', #16335, #3835, #11232, .T. ) ;
#12121=AXIS2_PLACEMENT_3D ( 'NONE', #18115, #310, #23887 ) ;
#12264=ADVANCED_FACE ( 'NONE', ( #24116 ), #10357, .T. ) ;
#12317=DIRECTION ( 'NONE',  ( 0.000000000000000000, 0.000000000000000000, 1.000000000000000000 ) ) ;
#12318=ADVANCED_FACE ( 'NONE', ( #12686 ), #9078, .T. ) ;
#12351=ORIENTED_EDGE ( 'NONE', *, *, #24955, .F. ) ;
#12368=DIRECTION ( 'NONE',  ( 0.000000000000000000, 3.491481338843134933E-15, 1.000000000000000000 ) ) ;
#12405=EDGE_CURVE ( 'NONE', #3835, #19999, #2599, .T. ) ;
#12430=VERTEX_POINT ( 'NONE', #1819 ) ;
#12486=AXIS2_PLACEMENT_3D ( 'NONE', #961, #24522, #4968 ) ;
#12530=AXIS2_PLACEMENT_3D ( 'NONE', #11994, #20082, #9678 ) ;
#12567=DIRECTION ( 'NONE',  ( 0.000000000000000000, 0.000000000000000000, -1.000000000000000000 ) ) ;
#12586=CARTESIAN_POINT ( 'NONE',  ( 43.81606138205700063, 36.92314894770293421, 79.37823623207322044 ) ) ;
#12590=CARTESIAN_POINT ( 'NONE',  ( 36.81465384343994884, 41.43850569188389699, 79.87823623207322044 ) ) ;
#12598=EDGE_CURVE ( 'NONE', #16335, #10282, #8785, .T. ) ;
#12607=CARTESIAN_POINT ( 'NONE',  ( 32.81606138205700773, 36.92314894770294131, 80.37823623207323465 ) ) ;
#12612=CARTESIAN_POINT ( 'NONE',  ( 45.81606138205700063, 36.92314894770293421, 79.37823623207323465 ) ) ;
#12636=CARTESIAN_POINT ( 'NONE',  ( 32.81606138205700773, 36.92314894770294131, 80.37823623207323465 ) ) ;
#12642=ORIENTED_EDGE ( 'NONE', *, *, #24380, .F. ) ;
#12652=CARTESIAN_POINT ( 'NONE',  ( 43.23147868389327897, 42.57231754924293909, 79.57823623207323749 ) ) ;
#12686=FACE_OUTER_BOUND ( 'NONE', #605, .T. ) ;
#12703=EDGE_LOOP ( 'NONE', ( #8075, #22847, #2907, #11842 ) ) ;
#12710=MECHANICAL_DESIGN_GEOMETRIC_PRESENTATION_REPRESENTATION('',(#22987),#6937);
#12723=DIRECTION ( 'NONE',  ( 1.000000000000000000, 6.938893903907222067E-15, 0.000000000000000000 ) ) ;
#12739=ADVANCED_FACE ( 'NONE', ( #24088 ), #20491, .T. ) ;
#12763=CARTESIAN_POINT ( 'NONE',  ( 32.81606138205700773, 36.92314894770293421, 79.37823623207323465 ) ) ;
#12764=AXIS2_PLACEMENT_3D ( 'NONE', #23754, #5995, #1980 ) ;
#12766=DIRECTION ( 'NONE',  ( 0.000000000000000000, 0.000000000000000000, 1.000000000000000000 ) ) ;
#12826=CYLINDRICAL_SURFACE ( 'NONE', #7592, 0.2000000000000057288 ) ;
#12827=EDGE_CURVE ( 'NONE', #23772, #1612, #6336, .T. ) ;
#12846=ORIENTED_EDGE ( 'NONE', *, *, #7743, .T. ) ;
#12848=VECTOR ( 'NONE', #23541, 1000.000000000000000 ) ;
#12864=DIRECTION ( 'NONE',  ( 1.734723475976805122E-16, 3.491481338843134933E-15, 1.000000000000000000 ) ) ;
#12875=ORIENTED_EDGE ( 'NONE', *, *, #22325, .T. ) ;
#12880=ORIENTED_EDGE ( 'NONE', *, *, #15581, .T. ) ;
#12887=CIRCLE ( 'NONE', #7943, 0.2314957320545540931 ) ;
#12891=DIRECTION ( 'NONE',  ( 0.000000000000000000, -6.938893903907222067E-15, -1.000000000000000000 ) ) ;
#12892=AXIS2_PLACEMENT_3D ( 'NONE', #23227, #7530, #2094 ) ;
#12896=DIRECTION ( 'NONE',  ( 0.000000000000000000, 1.000000000000000000, -3.469446951953613400E-15 ) ) ;
#12902=DIRECTION ( 'NONE',  ( 0.000000000000000000, 0.000000000000000000, -1.000000000000000000 ) ) ;
#12920=DIRECTION ( 'NONE',  ( 0.000000000000000000, 1.000000000000000000, 0.000000000000000000 ) ) ;
#12932=VERTEX_POINT ( 'NONE', #1416 ) ;
#12934=FACE_OUTER_BOUND ( 'NONE', #7952, .T. ) ;
#12952=ORIENTED_EDGE ( 'NONE', *, *, #25366, .F. ) ;
#12970=CARTESIAN_POINT ( 'NONE',  ( 36.81465384343994884, 41.90149715599300606, 79.87823623207322044 ) ) ;
#12974=EDGE_CURVE ( 'NONE', #24574, #1612, #17140, .T. ) ;
#12984=DIRECTION ( 'NONE',  ( 0.000000000000000000, 3.469446951953613400E-15, 1.000000000000000000 ) ) ;
#12986=VERTEX_POINT ( 'NONE', #11602 ) ;
#12996=CARTESIAN_POINT ( 'NONE',  ( 43.81606138205700063, 36.92314894770294131, 81.37823623207324886 ) ) ;
#13027=ORIENTED_EDGE ( 'NONE', *, *, #17919, .T. ) ;
#13113=EDGE_LOOP ( 'NONE', ( #10032, #5175, #6678, #10120 ) ) ;
#13115=DIRECTION ( 'NONE',  ( 0.000000000000000000, 0.000000000000000000, -1.000000000000000000 ) ) ;
#13125=DIRECTION ( 'NONE',  ( 0.000000000000000000, 1.000000000000000000, 0.000000000000000000 ) ) ;
#13149=CARTESIAN_POINT ( 'NONE',  ( 36.81465384343994884, 41.90149715599300606, 79.37823623207322044 ) ) ;
#13177=VECTOR ( 'NONE', #8782, 1000.000000000000000 ) ;
#13193=EDGE_CURVE ( 'NONE', #2757, #24470, #17040, .T. ) ;
#13227=AXIS2_PLACEMENT_3D ( 'NONE', #840, #5118, #14517 ) ;
#13228=ORIENTED_EDGE ( 'NONE', *, *, #5627, .T. ) ;
#13240=ORIENTED_EDGE ( 'NONE', *, *, #12405, .F. ) ;
#13243=EDGE_CURVE ( 'NONE', #23789, #9136, #4693, .T. ) ;
#13257=ORIENTED_EDGE ( 'NONE', *, *, #6867, .T. ) ;
#13271=VECTOR ( 'NONE', #3959, 1000.000000000000000 ) ;
#13272=EDGE_CURVE ( 'NONE', #23504, #17769, #9604, .T. ) ;
#13275=DIRECTION ( 'NONE',  ( -0.000000000000000000, -3.469446951953613400E-15, -1.000000000000000000 ) ) ;
#13280=CIRCLE ( 'NONE', #11223, 0.5000000000000004441 ) ;
#13330=CARTESIAN_POINT ( 'NONE',  ( 36.81465384343994884, 42.57231754924293909, 79.37823623207320622 ) ) ;
#13335=AXIS2_PLACEMENT_3D ( 'NONE', #16475, #18428, #757 ) ;
#13351=( NAMED_UNIT ( * ) SI_UNIT ( $, .STERADIAN. ) SOLID_ANGLE_UNIT ( ) );
#13355=AXIS2_PLACEMENT_3D ( 'NONE', #20390, #16009, #24230 ) ;
#13358=EDGE_LOOP ( 'NONE', ( #14739, #2941, #810, #1364 ) ) ;
#13465=( NAMED_UNIT ( * ) SI_UNIT ( $, .STERADIAN. ) SOLID_ANGLE_UNIT ( ) );
#13500=CARTESIAN_POINT ( 'NONE',  ( 32.81606138205700773, 35.92314894770293421, 79.37823623207323465 ) ) ;
#13525=CIRCLE ( 'NONE', #7344, 0.2000000000000057288 ) ;
#13580=CARTESIAN_POINT ( 'NONE',  ( 45.61606138205700489, 2.823374736507280597E-13, 81.37823623207336254 ) ) ;
#13606=ADVANCED_FACE ( 'NONE', ( #6386 ), #4450, .T. ) ;
#13607=DIRECTION ( 'NONE',  ( 6.938893903907221278E-15, -1.000000000000000000, 0.000000000000000000 ) ) ;
#13615=DIRECTION ( 'NONE',  ( -1.734723475976805122E-16, -3.491481338843134933E-15, -1.000000000000000000 ) ) ;
#13616=VERTEX_POINT ( 'NONE', #187 ) ;
#13633=ADVANCED_FACE ( 'NONE', ( #8065 ), #17983, .F. ) ;
#13651=EDGE_CURVE ( 'NONE', #21293, #3785, #17398, .T. ) ;
#13653=FACE_OUTER_BOUND ( 'NONE', #17452, .T. ) ;
#13704=ADVANCED_FACE ( 'NONE', ( #7143 ), #10884, .F. ) ;
#13724=DIRECTION ( 'NONE',  ( -1.000000000000000000, -0.000000000000000000, 0.000000000000000000 ) ) ;
#13759=DIRECTION ( 'NONE',  ( 0.000000000000000000, 0.000000000000000000, -1.000000000000000000 ) ) ;
#13779=FACE_OUTER_BOUND ( 'NONE', #14962, .T. ) ;
#13798=ORIENTED_EDGE ( 'NONE', *, *, #9367, .T. ) ;
#13846=VERTEX_POINT ( 'NONE', #13330 ) ;
#13876=CARTESIAN_POINT ( 'NONE',  ( 39.81746892067405952, 40.95934826813394380, 79.52109337493035923 ) ) ;
#13955=EDGE_LOOP ( 'NONE', ( #13987, #5395, #24658, #23942 ) ) ;
#13957=FACE_OUTER_BOUND ( 'NONE', #23760, .T. ) ;
#13987=ORIENTED_EDGE ( 'NONE', *, *, #13243, .T. ) ;
#13993=VERTEX_POINT ( 'NONE', #23475 ) ;
#14004=ORIENTED_EDGE ( 'NONE', *, *, #17764, .T. ) ;
#14022=CIRCLE ( 'NONE', #15668, 2.000000000000001776 ) ;
#14061=CIRCLE ( 'NONE', #4613, 2.000000000000001776 ) ;
#14075=AXIS2_PLACEMENT_3D ( 'NONE', #14811, #9163, #12896 ) ;
#14102=AXIS2_PLACEMENT_3D ( 'NONE', #7058, #3315, #736 ) ;
#14144=CIRCLE ( 'NONE', #21129, 0.2000000000000057288 ) ;
#14192=CARTESIAN_POINT ( 'NONE',  ( 32.81606138205700773, 44.92314894770294131, 80.37823623207322044 ) ) ;
#14249=DIRECTION ( 'NONE',  ( 1.734723475976805122E-16, 3.491481338843134933E-15, 1.000000000000000000 ) ) ;
#14278=DIRECTION ( 'NONE',  ( -0.000000000000000000, -3.469446951953613400E-15, -1.000000000000000000 ) ) ;
#14288=LINE ( 'NONE', #16086, #15186 ) ;
#14297=EDGE_CURVE ( 'NONE', #23482, #22567, #15701, .T. ) ;
#14300=AXIS2_PLACEMENT_3D ( 'NONE', #16507, #15089, #12920 ) ;
#14303=AXIS2_PLACEMENT_3D ( 'NONE', #2671, #12864, #24687 ) ;
#14335=CARTESIAN_POINT ( 'NONE',  ( 30.81606138205700418, 36.92314894770293421, 79.37823623207323465 ) ) ;
#14350=CARTESIAN_POINT ( 'NONE',  ( 45.81606138205700063, 46.72314894770294558, 81.17823623207318917 ) ) ;
#14377=ORIENTED_EDGE ( 'NONE', *, *, #24955, .T. ) ;
#14385=DIRECTION ( 'NONE',  ( 0.000000000000000000, 3.469446951953613400E-15, 1.000000000000000000 ) ) ;
#14386=EDGE_CURVE ( 'NONE', #9404, #23789, #7717, .T. ) ;
#14390=DIRECTION ( 'NONE',  ( 0.000000000000000000, 3.469446951953613400E-15, 1.000000000000000000 ) ) ;
#14455=CARTESIAN_POINT ( 'NONE',  ( 33.40064408022072939, 41.67000142393845152, 79.87823623207322044 ) ) ;
#14462=CARTESIAN_POINT ( 'NONE',  ( 0.000000000000000000, 46.72314894770294558, 81.37823623207320622 ) ) ;
#14476=CARTESIAN_POINT ( 'NONE',  ( 32.81606138205700773, 46.72314894770294558, 81.17823623207320338 ) ) ;
#14486=ORIENTED_EDGE ( 'NONE', *, *, #7973, .T. ) ;
#14503=ORIENTED_EDGE ( 'NONE', *, *, #7743, .F. ) ;
#14517=DIRECTION ( 'NONE',  ( 0.000000000000000000, 0.000000000000000000, -1.000000000000000000 ) ) ;
#14549=DIRECTION ( 'NONE',  ( -0.000000000000000000, -3.469446951953613400E-15, -1.000000000000000000 ) ) ;
#14554=CYLINDRICAL_SURFACE ( 'NONE', #13335, 1.000000000000000888 ) ;
#14558=DIRECTION ( 'NONE',  ( -1.000000000000000000, -0.000000000000000000, 0.000000000000000000 ) ) ;
#14624=EDGE_CURVE ( 'NONE', #23772, #9515, #4739, .T. ) ;
#14647=CARTESIAN_POINT ( 'NONE',  ( 39.81746892067405952, 41.67000142393845152, 79.52109337493035923 ) ) ;
#14655=CARTESIAN_POINT ( 'NONE',  ( 30.81606138205700418, 36.92314894770294131, 80.37823623207322044 ) ) ;
#14664=UNCERTAINTY_MEASURE_WITH_UNIT (LENGTH_MEASURE( 1.000000000000000082E-05 ), #11413, 'distance_accuracy_value', 'NONE');
#14690=DIRECTION ( 'NONE',  ( 0.000000000000000000, 1.000000000000000000, 0.000000000000000000 ) ) ;
#14726=EDGE_CURVE ( 'NONE', #10123, #24470, #15299, .T. ) ;
#14731=EDGE_LOOP ( 'NONE', ( #11051, #21985, #13240, #3691 ) ) ;
#14739=ORIENTED_EDGE ( 'NONE', *, *, #11713, .T. ) ;
#14745=ADVANCED_FACE ( 'NONE', ( #6798 ), #849, .T. ) ;
#14795=LINE ( 'NONE', #1508, #24652 ) ;
#14811=CARTESIAN_POINT ( 'NONE',  ( 43.81606138205700063, 36.92314894770294131, 80.37823623207323465 ) ) ;
#14817=DIRECTION ( 'NONE',  ( -0.000000000000000000, -3.469446951953613400E-15, -1.000000000000000000 ) ) ;
#14831=FACE_OUTER_BOUND ( 'NONE', #3849, .T. ) ;
#14871=DIRECTION ( 'NONE',  ( 0.000000000000000000, 0.000000000000000000, 1.000000000000000000 ) ) ;
#14903=CARTESIAN_POINT ( 'NONE',  ( 36.81465384343994884, 40.76768529863396395, 79.57823623207323749 ) ) ;
#14918=EDGE_CURVE ( 'NONE', #12986, #19369, #23553, .T. ) ;
#14942=DIRECTION ( 'NONE',  ( 1.000000000000000000, 0.000000000000000000, 0.000000000000000000 ) ) ;
#14948=EDGE_CURVE ( 'NONE', #16335, #1085, #15913, .T. ) ;
#14955=AXIS2_PLACEMENT_3D ( 'NONE', #10706, #4762, #2691 ) ;
#14962=EDGE_LOOP ( 'NONE', ( #11958, #16123, #14486, #12880, #13027, #3690, #1280, #2049 ) ) ;
#15055=EDGE_LOOP ( 'NONE', ( #3482, #501, #20157, #14503 ) ) ;
#15078=VERTEX_POINT ( 'NONE', #18122 ) ;
#15089=DIRECTION ( 'NONE',  ( -0.000000000000000000, -3.469446951953613400E-15, -1.000000000000000000 ) ) ;
#15115=ORIENTED_EDGE ( 'NONE', *, *, #18942, .F. ) ;
#15122=FACE_OUTER_BOUND ( 'NONE', #5599, .T. ) ;
#15133=ORIENTED_EDGE ( 'NONE', *, *, #4566, .T. ) ;
#15151=EDGE_CURVE ( 'NONE', #15078, #1612, #6286, .T. ) ;
#15158=CARTESIAN_POINT ( 'NONE',  ( 36.81465384343994884, 41.67000142393845152, 79.52109337493035923 ) ) ;
#15165=ADVANCED_FACE ( 'NONE', ( #10256 ), #18366, .T. ) ;
#15186=VECTOR ( 'NONE', #2296, 1000.000000000000000 ) ;
#15210=ORIENTED_EDGE ( 'NONE', *, *, #2154, .T. ) ;
#15227=CARTESIAN_POINT ( 'NONE',  ( 39.81746892067405952, 41.90149715599300606, 79.87823623207322044 ) ) ;
#15255=SURFACE_STYLE_USAGE ( .BOTH. , #25020 ) ;
#15263=AXIS2_PLACEMENT_3D ( 'NONE', #12763, #6947, #24704 ) ;
#15267=AXIS2_PLACEMENT_3D ( 'NONE', #23123, #25302, #21456 ) ;
#15299=CIRCLE ( 'NONE', #17365, 0.7106531558045068309 ) ;
#15303=AXIS2_PLACEMENT_3D ( 'NONE', #5026, #14942, #24578 ) ;
#15330=AXIS2_PLACEMENT_3D ( 'NONE', #4499, #20950, #16697 ) ;
#15396=DIRECTION ( 'NONE',  ( -0.000000000000000000, -3.469446951953613400E-15, -1.000000000000000000 ) ) ;
#15398=EDGE_CURVE ( 'NONE', #2345, #13616, #25195, .T. ) ;
#15416=ORIENTED_EDGE ( 'NONE', *, *, #11568, .T. ) ;
#15439=ORIENTED_EDGE ( 'NONE', *, *, #17615, .F. ) ;
#15441=EDGE_CURVE ( 'NONE', #9125, #9136, #165, .T. ) ;
#15444=EDGE_CURVE ( 'NONE', #23482, #24470, #19064, .T. ) ;
#15473=LINE ( 'NONE', #15735, #22227 ) ;
#15477=FACE_OUTER_BOUND ( 'NONE', #5222, .T. ) ;
#15496=ORIENTED_EDGE ( 'NONE', *, *, #9857, .T. ) ;
#15505=ORIENTED_EDGE ( 'NONE', *, *, #15444, .T. ) ;
#15507=CIRCLE ( 'NONE', #1505, 2.000000000000001776 ) ;
#15522=ORIENTED_EDGE ( 'NONE', *, *, #8106, .T. ) ;
#15532=ORIENTED_EDGE ( 'NONE', *, *, #14624, .F. ) ;
#15567=ORIENTED_EDGE ( 'NONE', *, *, #19038, .F. ) ;
#15581=EDGE_CURVE ( 'NONE', #3785, #19999, #10483, .T. ) ;
#15599=VECTOR ( 'NONE', #23599, 1000.000000000000000 ) ;
#15608=ADVANCED_FACE ( 'NONE', ( #13957 ), #10222, .T. ) ;
#15629=ORIENTED_EDGE ( 'NONE', *, *, #23724, .T. ) ;
#15662=FACE_OUTER_BOUND ( 'NONE', #6250, .T. ) ;
#15668=AXIS2_PLACEMENT_3D ( 'NONE', #22408, #14549, #7074 ) ;
#15701=CIRCLE ( 'NONE', #6263, 0.9023161253044892360 ) ;
#15717=ORIENTED_EDGE ( 'NONE', *, *, #5792, .T. ) ;
#15729=DIRECTION ( 'NONE',  ( 0.000000000000000000, 0.000000000000000000, 1.000000000000000000 ) ) ;
#15733=CIRCLE ( 'NONE', #15303, 0.2000000000000057288 ) ;
#15735=CARTESIAN_POINT ( 'NONE',  ( 30.81606138205700418, 36.92314894770294131, 80.37823623207323465 ) ) ;
#15743=AXIS2_PLACEMENT_3D ( 'NONE', #11799, #15396, #19636 ) ;
#15754=CARTESIAN_POINT ( 'NONE',  ( 44.81606138205700063, 36.92314894770293421, 79.37823623207323465 ) ) ;
#15761=DIRECTION ( 'NONE',  ( 0.000000000000000000, 3.469446951953613400E-15, 1.000000000000000000 ) ) ;
#15768=AXIS2_PLACEMENT_3D ( 'NONE', #10606, #6603, #15882 ) ;
#15779=AXIS2_PLACEMENT_3D ( 'NONE', #12652, #18438, #12902 ) ;
#15792=TOROIDAL_SURFACE ( 'NONE', #23530, 0.2314957320545545372, 0.5000000000000000000 ) ;
#15829=DIRECTION ( 'NONE',  ( 0.000000000000000000, -1.000000000000000000, 3.469446951953613794E-15 ) ) ;
#15857=DIRECTION ( 'NONE',  ( 0.000000000000000000, 3.469446951953613400E-15, 1.000000000000000000 ) ) ;
#15882=DIRECTION ( 'NONE',  ( 0.000000000000000000, -1.000000000000000000, 6.938893903907222067E-15 ) ) ;
#15887=CARTESIAN_POINT ( 'NONE',  ( 44.81606138205700063, 44.92314894770293421, 79.37823623207320622 ) ) ;
#15913=LINE ( 'NONE', #10007, #3387 ) ;
#15952=PLANE ( 'NONE',  #16545 ) ;
#15962=EDGE_LOOP ( 'NONE', ( #17736, #10561, #18565, #17830 ) ) ;
#15970=LINE ( 'NONE', #2192, #22428 ) ;
#16001=CIRCLE ( 'NONE', #784, 0.9023161253044892360 ) ;
#16008=AXIS2_PLACEMENT_3D ( 'NONE', #1780, #13275, #21127 ) ;
#16009=DIRECTION ( 'NONE',  ( 1.734723475976805122E-16, 3.491481338843134933E-15, 1.000000000000000000 ) ) ;
#16011=CARTESIAN_POINT ( 'NONE',  ( 32.81606138205700773, 44.92314894770294131, 81.17823623207320338 ) ) ;
#16062=CARTESIAN_POINT ( 'NONE',  ( 43.81606138205700063, 44.92314894770294131, 80.37823623207322044 ) ) ;
#16067=DIRECTION ( 'NONE',  ( 0.000000000000000000, 1.000000000000000000, -3.469446951953613400E-15 ) ) ;
#16081=DIRECTION ( 'NONE',  ( 0.000000000000000000, 0.000000000000000000, 1.000000000000000000 ) ) ;
#16086=CARTESIAN_POINT ( 'NONE',  ( 33.40064408022072939, 42.38065457974295924, 79.52109337493037344 ) ) ;
#16104=FACE_OUTER_BOUND ( 'NONE', #18600, .T. ) ;
#16123=ORIENTED_EDGE ( 'NONE', *, *, #15441, .T. ) ;
#16130=ORIENTED_EDGE ( 'NONE', *, *, #6786, .F. ) ;
#16192=CARTESIAN_POINT ( 'NONE',  ( 44.81606138205700063, 36.92314894770293421, 80.37823623207323465 ) ) ;
#16213=CARTESIAN_POINT ( 'NONE',  ( 33.40064408022072939, 40.76768529863396395, 79.57823623207325170 ) ) ;
#16246=AXIS2_PLACEMENT_3D ( 'NONE', #9026, #19062, #22912 ) ;
#16301=FACE_OUTER_BOUND ( 'NONE', #941, .T. ) ;
#16305=EDGE_CURVE ( 'NONE', #1848, #8440, #11282, .T. ) ;
#16308=EDGE_CURVE ( 'NONE', #1085, #22152, #145, .T. ) ;
#16321=ADVANCED_FACE ( 'NONE', ( #6955 ), #14554, .T. ) ;
#16335=VERTEX_POINT ( 'NONE', #22412 ) ;
#16364=AXIS2_PLACEMENT_3D ( 'NONE', #17464, #19381, #3285 ) ;
#16392=CARTESIAN_POINT ( 'NONE',  ( 43.23147868389327897, 42.38065457974295924, 79.52109337493035923 ) ) ;
#16435=DIRECTION ( 'NONE',  ( 0.000000000000000000, 3.469446951953613400E-15, 1.000000000000000000 ) ) ;
#16458=DIRECTION ( 'NONE',  ( -1.000000000000000000, 0.000000000000000000, 0.000000000000000000 ) ) ;
#16475=CARTESIAN_POINT ( 'NONE',  ( -3.469446951953610245E-16, 35.92314894770294131, 80.37823623207323465 ) ) ;
#16482=CARTESIAN_POINT ( 'NONE',  ( 45.61606138205700489, 36.92314894770294131, 81.37823623207324886 ) ) ;
#16507=CARTESIAN_POINT ( 'NONE',  ( 43.23147868389327897, 41.67000142393845152, 79.52109337493035923 ) ) ;
#16520=CARTESIAN_POINT ( 'NONE',  ( 39.81746892067405952, 41.67000142393845152, 79.37823623207322044 ) ) ;
#16524=DIRECTION ( 'NONE',  ( 1.000000000000000000, 0.000000000000000000, 0.000000000000000000 ) ) ;
#16545=AXIS2_PLACEMENT_3D ( 'NONE', #4747, #614, #12368 ) ;
#16559=CARTESIAN_POINT ( 'NONE',  ( 43.81606138205700063, 44.92314894770294131, 80.37823623207322044 ) ) ;
#16567=DIRECTION ( 'NONE',  ( -0.000000000000000000, -3.469446951953613400E-15, -1.000000000000000000 ) ) ;
#16570=DIRECTION ( 'NONE',  ( 0.000000000000000000, 3.469446951953613400E-15, 1.000000000000000000 ) ) ;
#16613=( GEOMETRIC_REPRESENTATION_CONTEXT ( 3 ) GLOBAL_UNCERTAINTY_ASSIGNED_CONTEXT ( ( #14664 ) ) GLOBAL_UNIT_ASSIGNED_CONTEXT ( ( #11413, #3537, #13351 ) ) REPRESENTATION_CONTEXT ( 'NONE', 'WORKASPACE' ) );
#16644=EDGE_LOOP ( 'NONE', ( #23343, #21931, #17246, #23755 ) ) ;
#16658=DIRECTION ( 'NONE',  ( 0.000000000000000000, 1.000000000000000000, -3.469446951953613794E-15 ) ) ;
#16697=DIRECTION ( 'NONE',  ( 0.000000000000000000, 0.000000000000000000, -1.000000000000000000 ) ) ;
#16716=DIRECTION ( 'NONE',  ( 0.000000000000000000, 3.469446951953613400E-15, 1.000000000000000000 ) ) ;
#16746=DIRECTION ( 'NONE',  ( 0.000000000000000000, 0.000000000000000000, 1.000000000000000000 ) ) ;
#16756=DIRECTION ( 'NONE',  ( 0.000000000000000000, -1.000000000000000000, 3.469446951953613794E-15 ) ) ;
#16799=AXIS2_PLACEMENT_3D ( 'NONE', #20693, #3029, #24786 ) ;
#16829=CARTESIAN_POINT ( 'NONE',  ( 33.40064408022072939, 41.43850569188389699, 79.87823623207322044 ) ) ;
#16832=CYLINDRICAL_SURFACE ( 'NONE', #13227, 0.5000000000000004441 ) ;
#16839=ORIENTED_EDGE ( 'NONE', *, *, #6086, .T. ) ;
#16845=CARTESIAN_POINT ( 'NONE',  ( 45.81606138205700063, 34.92314894770294131, 81.17823623207323180 ) ) ;
#16857=CARTESIAN_POINT ( 'NONE',  ( 33.40064408022072939, 41.67000142393845152, 79.52109337493035923 ) ) ;
#16866=VECTOR ( 'NONE', #22344, 1000.000000000000000 ) ;
#16924=DIRECTION ( 'NONE',  ( 0.000000000000000000, -3.469446951953613400E-15, -1.000000000000000000 ) ) ;
#16946=ORIENTED_EDGE ( 'NONE', *, *, #11241, .T. ) ;
#16958=DIRECTION ( 'NONE',  ( 6.938893903907221278E-15, -1.000000000000000000, 0.000000000000000000 ) ) ;
#16961=AXIS2_PLACEMENT_3D ( 'NONE', #352, #16458, #16081 ) ;
#16984=AXIS2_PLACEMENT_3D ( 'NONE', #17235, #5897, #13759 ) ;
#17027=AXIS2_PLACEMENT_3D ( 'NONE', #1056, #24112, #2725 ) ;
#17040=CIRCLE ( 'NONE', #12530, 0.5000000000000004441 ) ;
#17046=CARTESIAN_POINT ( 'NONE',  ( 43.81606138205700063, 45.92314894770293421, 79.37823623207320622 ) ) ;
#17055=APPLICATION_CONTEXT ( 'automotive_design' ) ;
#17076=( NAMED_UNIT ( * ) PLANE_ANGLE_UNIT ( ) SI_UNIT ( $, .RADIAN. ) );
#17115=ADVANCED_FACE ( 'NONE', ( #20263 ), #22445, .T. ) ;
#17140=LINE ( 'NONE', #24718, #10457 ) ;
#17158=AXIS2_PLACEMENT_3D ( 'NONE', #17421, #22955, #11506 ) ;
#17166=DIRECTION ( 'NONE',  ( 1.000000000000000000, 0.000000000000000000, -0.000000000000000000 ) ) ;
#17198=TOROIDAL_SURFACE ( 'NONE', #9388, 1.800000000000000044, 0.2000000000000000111 ) ;
#17202=VERTEX_POINT ( 'NONE', #2476 ) ;
#17211=EDGE_CURVE ( 'NONE', #9789, #13993, #2533, .T. ) ;
#17218=AXIS2_PLACEMENT_3D ( 'NONE', #16559, #22240, #2766 ) ;
#17232=AXIS2_PLACEMENT_3D ( 'NONE', #17974, #6242, #8308 ) ;
#17235=CARTESIAN_POINT ( 'NONE',  ( 32.81606138205700773, 45.92314894770293421, 80.37823623207322044 ) ) ;
#17246=ORIENTED_EDGE ( 'NONE', *, *, #14386, .F. ) ;
#17303=EDGE_CURVE ( 'NONE', #21293, #23789, #14061, .T. ) ;
#17322=ORIENTED_EDGE ( 'NONE', *, *, #6265, .F. ) ;
#17342=CARTESIAN_POINT ( 'NONE',  ( 43.81606138205700063, 34.92314894770294131, 80.37823623207323465 ) ) ;
#17365=AXIS2_PLACEMENT_3D ( 'NONE', #14647, #8483, #24425 ) ;
#17370=CIRCLE ( 'NONE', #11220, 0.2000000000000057288 ) ;
#17386=CARTESIAN_POINT ( 'NONE',  ( 31.81606138205700418, 36.92314894770293421, 79.37823623207323465 ) ) ;
#17398=CIRCLE ( 'NONE', #12121, 0.2000000000000057288 ) ;
#17412=DIRECTION ( 'NONE',  ( 0.000000000000000000, -3.469446951953613400E-15, -1.000000000000000000 ) ) ;
#17421=CARTESIAN_POINT ( 'NONE',  ( 43.23147868389327897, 41.67000142393845152, 79.87823623207322044 ) ) ;
#17431=DIRECTION ( 'NONE',  ( 0.000000000000000000, 1.000000000000000000, 0.000000000000000000 ) ) ;
#17449=DIRECTION ( 'NONE',  ( 0.000000000000000000, 0.000000000000000000, -1.000000000000000000 ) ) ;
#17452=EDGE_LOOP ( 'NONE', ( #13798, #3622, #21562, #7451 ) ) ;
#17462=MECHANICAL_DESIGN_GEOMETRIC_PRESENTATION_REPRESENTATION('',(#19923),#24023);
#17464=CARTESIAN_POINT ( 'NONE',  ( 43.81606138205700063, 44.92314894770293421, 79.37823623207320622 ) ) ;
#17486=CARTESIAN_POINT ( 'NONE',  ( 43.81606138205700063, 34.92314894770293421, 80.37823623207323465 ) ) ;
#17498=ADVANCED_FACE ( 'NONE', ( #16104 ), #22714, .T. ) ;
#17500=LINE ( 'NONE', #9519, #13271 ) ;
#17589=ORIENTED_EDGE ( 'NONE', *, *, #24661, .F. ) ;
#17615=EDGE_CURVE ( 'NONE', #2345, #3400, #15733, .T. ) ;
#17616=EDGE_CURVE ( 'NONE', #10282, #11605, #24843, .T. ) ;
#17622=AXIS2_PLACEMENT_3D ( 'NONE', #6068, #21651, #15729 ) ;
#17628=ADVANCED_FACE ( 'NONE', ( #10710 ), #21488, .T. ) ;
#17634=ORIENTED_EDGE ( 'NONE', *, *, #11646, .F. ) ;
#17736=ORIENTED_EDGE ( 'NONE', *, *, #12405, .T. ) ;
#17739=TOROIDAL_SURFACE ( 'NONE', #11570, 0.9023161253044896801, 0.2000000000000000111 ) ;
#17755=ORIENTED_EDGE ( 'NONE', *, *, #2154, .F. ) ;
#17764=EDGE_CURVE ( 'NONE', #13846, #12986, #17370, .T. ) ;
#17769=VERTEX_POINT ( 'NONE', #8475 ) ;
#17772=ADVANCED_FACE ( 'NONE', ( #2528 ), #10388, .T. ) ;
#17813=ADVANCED_FACE ( 'NONE', ( #6534 ), #485, .T. ) ;
#17827=DIRECTION ( 'NONE',  ( 8.758115402030106693E-47, -1.000000000000000000, 3.469446951953613400E-15 ) ) ;
#17830=ORIENTED_EDGE ( 'NONE', *, *, #21704, .F. ) ;
#17868=LINE ( 'NONE', #17486, #21025 ) ;
#17898=ORIENTED_EDGE ( 'NONE', *, *, #17764, .F. ) ;
#17919=EDGE_CURVE ( 'NONE', #19999, #10282, #7927, .T. ) ;
#17920=CARTESIAN_POINT ( 'NONE',  ( 43.23147868389327897, 41.43850569188389699, 79.87823623207322044 ) ) ;
#17955=DIRECTION ( 'NONE',  ( -0.000000000000000000, -3.469446951953613400E-15, -1.000000000000000000 ) ) ;
#17967=DIRECTION ( 'NONE',  ( -0.000000000000000000, -3.469446951953613400E-15, -1.000000000000000000 ) ) ;
#17974=CARTESIAN_POINT ( 'NONE',  ( 39.81746892067405952, 41.43850569188389699, 79.37823623207322044 ) ) ;
#17983=CYLINDRICAL_SURFACE ( 'NONE', #2983, 0.5000000000000004441 ) ;
#18108=CIRCLE ( 'NONE', #6562, 0.9023161253044892360 ) ;
#18115=CARTESIAN_POINT ( 'NONE',  ( 43.81606138205700063, 46.72314894770294558, 81.17823623207318917 ) ) ;
#18122=CARTESIAN_POINT ( 'NONE',  ( 43.81606138205700063, 35.12314894770293705, 81.37823623207324886 ) ) ;
#18143=ORIENTED_EDGE ( 'NONE', *, *, #25442, .T. ) ;
#18155=FACE_OUTER_BOUND ( 'NONE', #5146, .T. ) ;
#18185=CARTESIAN_POINT ( 'NONE',  ( 43.23147868389327897, 42.38065457974295924, 79.52109337493037344 ) ) ;
#18211=CARTESIAN_POINT ( 'NONE',  ( 32.81606138205700773, 35.12314894770294416, 81.17823623207323180 ) ) ;
#18215=ORIENTED_EDGE ( 'NONE', *, *, #4239, .F. ) ;
#18218=EDGE_CURVE ( 'NONE', #15078, #9125, #22116, .T. ) ;
#18224=ADVANCED_FACE ( 'NONE', ( #20341 ), #18781, .T. ) ;
#18226=AXIS2_PLACEMENT_3D ( 'NONE', #23551, #11472, #2040 ) ;
#18240=UNCERTAINTY_MEASURE_WITH_UNIT (LENGTH_MEASURE( 1.000000000000000082E-05 ), #19502, 'distance_accuracy_value', 'NONE');
#18271=ORIENTED_EDGE ( 'NONE', *, *, #11580, .F. ) ;
#18273=DIRECTION ( 'NONE',  ( -0.000000000000000000, -3.469446951953613400E-15, -1.000000000000000000 ) ) ;
#18291=AXIS2_PLACEMENT_3D ( 'NONE', #22441, #20259, #6602 ) ;
#18305=FACE_OUTER_BOUND ( 'NONE', #4212, .T. ) ;
#18354=ORIENTED_EDGE ( 'NONE', *, *, #1385, .T. ) ;
#18356=ORIENTED_EDGE ( 'NONE', *, *, #15151, .F. ) ;
#18366=CYLINDRICAL_SURFACE ( 'NONE', #20680, 2.000000000000001776 ) ;
#18385=DIRECTION ( 'NONE',  ( 0.000000000000000000, 0.000000000000000000, 1.000000000000000000 ) ) ;
#18426=ORIENTED_EDGE ( 'NONE', *, *, #25366, .T. ) ;
#18428=DIRECTION ( 'NONE',  ( 1.000000000000000000, 0.000000000000000000, 0.000000000000000000 ) ) ;
#18438=DIRECTION ( 'NONE',  ( 1.000000000000000000, 0.000000000000000000, 0.000000000000000000 ) ) ;
#18446=DIRECTION ( 'NONE',  ( 0.000000000000000000, 3.469446951953613400E-15, 1.000000000000000000 ) ) ;
#18488=EDGE_LOOP ( 'NONE', ( #7295, #1138, #20854, #19124 ) ) ;
#18507=DIRECTION ( 'NONE',  ( 0.000000000000000000, -1.000000000000000000, 3.469446951953613400E-15 ) ) ;
#18565=ORIENTED_EDGE ( 'NONE', *, *, #13651, .F. ) ;
#18600=EDGE_LOOP ( 'NONE', ( #9049, #10302, #2763, #24399 ) ) ;
#18644=DIRECTION ( 'NONE',  ( 0.000000000000000000, 1.000000000000000000, 0.000000000000000000 ) ) ;
#18647=DIRECTION ( 'NONE',  ( 1.000000000000000000, 0.000000000000000000, 0.000000000000000000 ) ) ;
#18661=DIRECTION ( 'NONE',  ( 1.000000000000000000, 0.000000000000000000, 0.000000000000000000 ) ) ;
#18759=EDGE_CURVE ( 'NONE', #5707, #235, #22365, .T. ) ;
#18781=CYLINDRICAL_SURFACE ( 'NONE', #14303, 2.000000000000001776 ) ;
#18798=EDGE_LOOP ( 'NONE', ( #9712, #5890, #17322, #18143 ) ) ;
#18812=LINE ( 'NONE', #6833, #13177 ) ;
#18843=CIRCLE ( 'NONE', #16364, 1.000000000000000888 ) ;
#18887=ORIENTED_EDGE ( 'NONE', *, *, #12095, .T. ) ;
#18890=FACE_OUTER_BOUND ( 'NONE', #13358, .T. ) ;
#18932=VECTOR ( 'NONE', #20349, 1000.000000000000000 ) ;
#18942=EDGE_CURVE ( 'NONE', #1848, #1711, #18843, .T. ) ;
#18960=ORIENTED_EDGE ( 'NONE', *, *, #14726, .T. ) ;
#19004=DIRECTION ( 'NONE',  ( -1.000000000000000000, 0.000000000000000000, 0.000000000000000000 ) ) ;
#19038=EDGE_CURVE ( 'NONE', #23504, #11694, #22131, .T. ) ;
#19062=DIRECTION ( 'NONE',  ( 1.000000000000000000, 0.000000000000000000, -0.000000000000000000 ) ) ;
#19064=CIRCLE ( 'NONE', #1755, 0.2000000000000057288 ) ;
#19124=ORIENTED_EDGE ( 'NONE', *, *, #19946, .T. ) ;
#19170=EDGE_LOOP ( 'NONE', ( #15133, #15496, #1393, #25466, #24597, #7501, #24802, #599 ) ) ;
#19209=AXIS2_PLACEMENT_3D ( 'NONE', #5570, #3503, #3890 ) ;
#19227=CYLINDRICAL_SURFACE ( 'NONE', #6945, 0.2000000000000057288 ) ;
#19237=VERTEX_POINT ( 'NONE', #13500 ) ;
#19256=FILL_AREA_STYLE_COLOUR ( '', #5523 ) ;
#19279=CIRCLE ( 'NONE', #8177, 2.000000000000001776 ) ;
#19283=AXIS2_PLACEMENT_3D ( 'NONE', #19355, #16924, #17431 ) ;
#19325=ORIENTED_EDGE ( 'NONE', *, *, #22162, .T. ) ;
#19355=CARTESIAN_POINT ( 'NONE',  ( 39.81746892067405952, 41.67000142393845152, 79.87823623207322044 ) ) ;
#19369=VERTEX_POINT ( 'NONE', #7968 ) ;
#19381=DIRECTION ( 'NONE',  ( -0.000000000000000000, -3.469446951953613400E-15, -1.000000000000000000 ) ) ;
#19383=AXIS2_PLACEMENT_3D ( 'NONE', #21337, #1493, #13115 ) ;
#19425=ORIENTED_EDGE ( 'NONE', *, *, #2006, .F. ) ;
#19469=ADVANCED_FACE ( 'NONE', ( #16301 ), #1984, .T. ) ;
#19481=ADVANCED_FACE ( 'NONE', ( #3963 ), #20092, .F. ) ;
#19495=EDGE_CURVE ( 'NONE', #11605, #9789, #5288, .T. ) ;
#19502=( LENGTH_UNIT ( ) NAMED_UNIT ( * ) SI_UNIT ( .MILLI., .METRE. ) );
#19515=( LENGTH_UNIT ( ) NAMED_UNIT ( * ) SI_UNIT ( .MILLI., .METRE. ) );
#19551=AXIS2_PLACEMENT_3D ( 'NONE', #19718, #17412, #3614 ) ;
#19586=ORIENTED_EDGE ( 'NONE', *, *, #15151, .T. ) ;
#19606=DIRECTION ( 'NONE',  ( 1.000000000000000000, 0.000000000000000000, 0.000000000000000000 ) ) ;
#19636=DIRECTION ( 'NONE',  ( 0.000000000000000000, 1.000000000000000000, 0.000000000000000000 ) ) ;
#19641=CARTESIAN_POINT ( 'NONE',  ( 32.81606138205700773, 46.92314894770294131, 80.37823623207322044 ) ) ;
#19708=CIRCLE ( 'NONE', #1602, 2.000000000000001776 ) ;
#19718=CARTESIAN_POINT ( 'NONE',  ( 43.23147868389327897, 41.67000142393845152, 79.87823623207322044 ) ) ;
#19729=CIRCLE ( 'NONE', #8635, 0.2314957320545540931 ) ;
#19733=DIRECTION ( 'NONE',  ( 0.000000000000000000, 1.000000000000000000, -0.000000000000000000 ) ) ;
#19744=LINE ( 'NONE', #15754, #4932 ) ;
#19821=EDGE_CURVE ( 'NONE', #10110, #10123, #765, .T. ) ;
#19892=CARTESIAN_POINT ( 'NONE',  ( 43.81606138205700063, 34.92314894770294131, 81.17823623207323180 ) ) ;
#19917=ORIENTED_EDGE ( 'NONE', *, *, #14948, .F. ) ;
#19918=CARTESIAN_POINT ( 'NONE',  ( 33.40064408022072939, 41.90149715599300606, 79.87823623207322044 ) ) ;
#19920=DIRECTION ( 'NONE',  ( 0.000000000000000000, 0.000000000000000000, -1.000000000000000000 ) ) ;
#19923=STYLED_ITEM ( 'NONE', ( #11298 ), #9253 ) ;
#19946=EDGE_CURVE ( 'NONE', #8440, #947, #5865, .T. ) ;
#19997=ORIENTED_EDGE ( 'NONE', *, *, #625, .F. ) ;
#19999=VERTEX_POINT ( 'NONE', #20400 ) ;
#20023=CARTESIAN_POINT ( 'NONE',  ( 32.81606138205700773, 46.92314894770294131, 80.37823623207322044 ) ) ;
#20048=FACE_OUTER_BOUND ( 'NONE', #13955, .T. ) ;
#20082=DIRECTION ( 'NONE',  ( -1.000000000000000000, 0.000000000000000000, 0.000000000000000000 ) ) ;
#20092=TOROIDAL_SURFACE ( 'NONE', #16799, 0.2314957320545545372, 0.5000000000000000000 ) ;
#20157=ORIENTED_EDGE ( 'NONE', *, *, #15398, .T. ) ;
#20163=CARTESIAN_POINT ( 'NONE',  ( 43.23147868389327897, 41.43850569188389699, 79.37823623207322044 ) ) ;
#20168=CARTESIAN_POINT ( 'NONE',  ( 30.81606138205700418, 46.92314894770294131, 81.17823623207320338 ) ) ;
#20198=ORIENTED_EDGE ( 'NONE', *, *, #12598, .F. ) ;
#20228=EDGE_CURVE ( 'NONE', #10110, #2757, #4882, .T. ) ;
#20234=CARTESIAN_POINT ( 'NONE',  ( 45.61606138205700489, 44.92314894770294131, 81.37823623207322044 ) ) ;
#20259=DIRECTION ( 'NONE',  ( -0.000000000000000000, -3.469446951953613400E-15, -1.000000000000000000 ) ) ;
#20263=FACE_OUTER_BOUND ( 'NONE', #16644, .T. ) ;
#20278=ADVANCED_FACE ( 'NONE', ( #21043 ), #19227, .T. ) ;
#20289=DIRECTION ( 'NONE',  ( 0.000000000000000000, -3.469446951953613400E-15, -1.000000000000000000 ) ) ;
#20293=VECTOR ( 'NONE', #8210, 1000.000000000000000 ) ;
#20341=FACE_OUTER_BOUND ( 'NONE', #18798, .T. ) ;
#20349=DIRECTION ( 'NONE',  ( -1.000000000000000000, 0.000000000000000000, 0.000000000000000000 ) ) ;
#20381=ORIENTED_EDGE ( 'NONE', *, *, #2372, .F. ) ;
#20390=CARTESIAN_POINT ( 'NONE',  ( 43.81606138205700063, 44.92314894770293421, 79.37823623207320622 ) ) ;
#20399=CARTESIAN_POINT ( 'NONE',  ( 31.01606138205699992, 46.92314894770294131, 81.17823623207318917 ) ) ;
#20400=CARTESIAN_POINT ( 'NONE',  ( 32.81606138205700773, 46.72314894770294558, 81.37823623207320622 ) ) ;
#20420=EDGE_CURVE ( 'NONE', #13993, #6274, #3896, .T. ) ;
#20423=DIRECTION ( 'NONE',  ( 8.758115402030106693E-47, -1.000000000000000000, 3.469446951953613400E-15 ) ) ;
#20451=DIRECTION ( 'NONE',  ( -1.734723475976805122E-16, -3.491481338843134933E-15, -1.000000000000000000 ) ) ;
#20491=CYLINDRICAL_SURFACE ( 'NONE', #15779, 0.2000000000000057288 ) ;
#20508=DIRECTION ( 'NONE',  ( 0.000000000000000000, 3.469446951953613400E-15, 1.000000000000000000 ) ) ;
#20515=DIRECTION ( 'NONE',  ( 1.000000000000000000, 0.000000000000000000, 0.000000000000000000 ) ) ;
#20556=FACE_OUTER_BOUND ( 'NONE', #22679, .T. ) ;
#20577=DIRECTION ( 'NONE',  ( -8.758115402030106693E-47, 1.000000000000000000, -3.469446951953613400E-15 ) ) ;
#20595=VECTOR ( 'NONE', #2380, 1000.000000000000000 ) ;
#20659=APPLICATION_CONTEXT ( 'automotive_design' ) ;
#20661=AXIS2_PLACEMENT_3D ( 'NONE', #14192, #10452, #8516 ) ;
#20680=AXIS2_PLACEMENT_3D ( 'NONE', #12586, #14249, #22093 ) ;
#20693=CARTESIAN_POINT ( 'NONE',  ( 43.23147868389327897, 41.67000142393845152, 79.37823623207322044 ) ) ;
#20697=PLANE ( 'NONE',  #1608 ) ;
#20713=LINE ( 'NONE', #16845, #5457 ) ;
#20730=EDGE_CURVE ( 'NONE', #10306, #17769, #16001, .T. ) ;
#20751=AXIS2_PLACEMENT_3D ( 'NONE', #23349, #21812, #17449 ) ;
#20768=ORIENTED_EDGE ( 'NONE', *, *, #14918, .F. ) ;
#20787=CARTESIAN_POINT ( 'NONE',  ( 33.40064408022072939, 41.43850569188389699, 79.37823623207322044 ) ) ;
#20854=ORIENTED_EDGE ( 'NONE', *, *, #251, .T. ) ;
#20856=PRODUCT_DEFINITION_CONTEXT ( 'detailed design', #20659, 'design' ) ;
#20863=DIRECTION ( 'NONE',  ( 0.000000000000000000, -1.000000000000000000, 6.938893903907221278E-15 ) ) ;
#20870=TOROIDAL_SURFACE ( 'NONE', #3569, 1.800000000000000044, 0.2000000000000000111 ) ;
#20892=PLANE ( 'NONE',  #22234 ) ;
#20930=ORIENTED_EDGE ( 'NONE', *, *, #7448, .T. ) ;
#20950=DIRECTION ( 'NONE',  ( 0.000000000000000000, -1.000000000000000000, 0.000000000000000000 ) ) ;
#21025=VECTOR ( 'NONE', #11816, 1000.000000000000000 ) ;
#21032=DIRECTION ( 'NONE',  ( 0.000000000000000000, 0.000000000000000000, -1.000000000000000000 ) ) ;
#21040=PRODUCT_CONTEXT ( 'NONE', #17055, 'mechanical' ) ;
#21043=FACE_OUTER_BOUND ( 'NONE', #22084, .T. ) ;
#21061=CARTESIAN_POINT ( 'NONE',  ( 33.40064408022072939, 42.57231754924293909, 79.57823623207322328 ) ) ;
#21099=AXIS2_PLACEMENT_3D ( 'NONE', #14903, #18647, #10548 ) ;
#21120=AXIS2_PLACEMENT_3D ( 'NONE', #519, #19733, #14 ) ;
#21127=DIRECTION ( 'NONE',  ( 0.000000000000000000, 1.000000000000000000, -3.469446951953613400E-15 ) ) ;
#21129=AXIS2_PLACEMENT_3D ( 'NONE', #9729, #3534, #1474 ) ;
#21136=ORIENTED_EDGE ( 'NONE', *, *, #20420, .T. ) ;
#21188=DIRECTION ( 'NONE',  ( 0.000000000000000000, 0.000000000000000000, -1.000000000000000000 ) ) ;
#21223=ORIENTED_EDGE ( 'NONE', *, *, #17303, .F. ) ;
#21225=EDGE_CURVE ( 'NONE', #23789, #23772, #14795, .T. ) ;
#21293=VERTEX_POINT ( 'NONE', #9866 ) ;
#21303=DIRECTION ( 'NONE',  ( 0.000000000000000000, 0.000000000000000000, 1.000000000000000000 ) ) ;
#21305=SURFACE_STYLE_FILL_AREA ( #24770 ) ;
#21326=ORIENTED_EDGE ( 'NONE', *, *, #23720, .F. ) ;
#21337=CARTESIAN_POINT ( 'NONE',  ( 33.40064408022072939, 41.90149715599300606, 79.37823623207322044 ) ) ;
#21360=ADVANCED_FACE ( 'NONE', ( #2364 ), #20870, .T. ) ;
#21363=CIRCLE ( 'NONE', #10271, 1.000000000000000888 ) ;
#21372=FACE_OUTER_BOUND ( 'NONE', #4879, .T. ) ;
#21399=DIRECTION ( 'NONE',  ( -1.734723475976805122E-16, -3.491481338843134933E-15, -1.000000000000000000 ) ) ;
#21404=CARTESIAN_POINT ( 'NONE',  ( 43.81606138205700063, 44.92314894770294131, 81.37823623207322044 ) ) ;
#21427=AXIS2_PLACEMENT_3D ( 'NONE', #16192, #16958, #12723 ) ;
#21456=DIRECTION ( 'NONE',  ( 0.000000000000000000, 0.000000000000000000, 1.000000000000000000 ) ) ;
#21472=AXIS2_PLACEMENT_3D ( 'NONE', #18211, #17166, #21032 ) ;
#21488=TOROIDAL_SURFACE ( 'NONE', #14075, 1.000000000000000000, 1.000000000000000000 ) ;
#21503=CARTESIAN_POINT ( 'NONE',  ( 45.81606138205700063, 36.92314894770294131, 80.37823623207323465 ) ) ;
#21528=LINE ( 'NONE', #7365, #5653 ) ;
#21531=VECTOR ( 'NONE', #5382, 1000.000000000000000 ) ;
#21562=ORIENTED_EDGE ( 'NONE', *, *, #6867, .F. ) ;
#21567=DIRECTION ( 'NONE',  ( 0.000000000000000000, 1.000000000000000000, 0.000000000000000000 ) ) ;
#21571=CARTESIAN_POINT ( 'NONE',  ( 43.23147868389327897, 40.95934826813394380, 79.52109337493037344 ) ) ;
#21631=ORIENTED_EDGE ( 'NONE', *, *, #3030, .F. ) ;
#21638=VERTEX_POINT ( 'NONE', #5965 ) ;
#21651=DIRECTION ( 'NONE',  ( -1.000000000000000000, 0.000000000000000000, 0.000000000000000000 ) ) ;
#21702=CYLINDRICAL_SURFACE ( 'NONE', #12764, 1.000000000000000888 ) ;
#21704=EDGE_CURVE ( 'NONE', #3835, #21293, #10211, .T. ) ;
#21729=ORIENTED_EDGE ( 'NONE', *, *, #7371, .T. ) ;
#21812=DIRECTION ( 'NONE',  ( 1.000000000000000000, 0.000000000000000000, 0.000000000000000000 ) ) ;
#21822=CARTESIAN_POINT ( 'NONE',  ( 43.81606138205700063, 36.92314894770294131, 80.37823623207323465 ) ) ;
#21857=ADVANCED_FACE ( 'NONE', ( #24342 ), #6468, .F. ) ;
#21869=DIRECTION ( 'NONE',  ( 0.000000000000000000, -1.000000000000000000, 3.491481338843134933E-15 ) ) ;
#21870=DIRECTION ( 'NONE',  ( 0.000000000000000000, 1.000000000000000000, 0.000000000000000000 ) ) ;
#21882=ORIENTED_EDGE ( 'NONE', *, *, #18218, .F. ) ;
#21886=DIRECTION ( 'NONE',  ( 0.000000000000000000, 1.000000000000000000, -3.469446951953613400E-15 ) ) ;
#21888=AXIS2_PLACEMENT_3D ( 'NONE', #22007, #20577, #8740 ) ;
#21925=VECTOR ( 'NONE', #25400, 1000.000000000000000 ) ;
#21931=ORIENTED_EDGE ( 'NONE', *, *, #17303, .T. ) ;
#21985=ORIENTED_EDGE ( 'NONE', *, *, #17919, .F. ) ;
#22007=CARTESIAN_POINT ( 'NONE',  ( 44.81606138205700063, 2.788239579249953820E-13, 80.37823623207336254 ) ) ;
#22084=EDGE_LOOP ( 'NONE', ( #18426, #16130, #14004, #23895 ) ) ;
#22093=DIRECTION ( 'NONE',  ( 0.000000000000000000, -1.000000000000000000, 6.938893903907222067E-15 ) ) ;
#22116=CIRCLE ( 'NONE', #24958, 1.800000000000002931 ) ;
#22131=CIRCLE ( 'NONE', #11036, 0.7106531558045068309 ) ;
#22133=CARTESIAN_POINT ( 'NONE',  ( 45.81606138205700063, 44.92314894770294131, 80.37823623207322044 ) ) ;
#22152=VERTEX_POINT ( 'NONE', #22267 ) ;
#22162=EDGE_CURVE ( 'NONE', #11694, #12986, #14288, .T. ) ;
#22189=ORIENTED_EDGE ( 'NONE', *, *, #17616, .F. ) ;
#22198=ORIENTED_EDGE ( 'NONE', *, *, #19821, .T. ) ;
#22225=ORIENTED_EDGE ( 'NONE', *, *, #23724, .F. ) ;
#22227=VECTOR ( 'NONE', #9820, 1000.000000000000000 ) ;
#22234=AXIS2_PLACEMENT_3D ( 'NONE', #9186, #11107, #22689 ) ;
#22237=DIRECTION ( 'NONE',  ( 0.000000000000000000, -1.000000000000000000, 0.000000000000000000 ) ) ;
#22239=EDGE_LOOP ( 'NONE', ( #1516, #17755, #15439, #2033 ) ) ;
#22240=DIRECTION ( 'NONE',  ( -0.000000000000000000, -3.469446951953613400E-15, -1.000000000000000000 ) ) ;
#22241=DIRECTION ( 'NONE',  ( 0.000000000000000000, -3.491481338843134933E-15, -1.000000000000000000 ) ) ;
#22251=AXIS2_PLACEMENT_3D ( 'NONE', #22530, #22791, #2811 ) ;
#22267=CARTESIAN_POINT ( 'NONE',  ( 31.81606138205700418, 44.92314894770293421, 79.37823623207320622 ) ) ;
#22318=DIRECTION ( 'NONE',  ( -1.000000000000000000, -0.000000000000000000, -0.000000000000000000 ) ) ;
#22325=EDGE_CURVE ( 'NONE', #24574, #7575, #774, .T. ) ;
#22344=DIRECTION ( 'NONE',  ( 1.000000000000000000, -0.000000000000000000, -0.000000000000000000 ) ) ;
#22349=ORIENTED_EDGE ( 'NONE', *, *, #3567, .F. ) ;
#22365=LINE ( 'NONE', #12970, #11448 ) ;
#22394=LINE ( 'NONE', #22133, #1730 ) ;
#22398=CIRCLE ( 'NONE', #20751, 0.2000000000000057288 ) ;
#22408=CARTESIAN_POINT ( 'NONE',  ( 32.81606138205700773, 36.92314894770294131, 81.17823623207323180 ) ) ;
#22412=CARTESIAN_POINT ( 'NONE',  ( 30.81606138205700418, 44.92314894770294131, 81.17823623207321759 ) ) ;
#22428=VECTOR ( 'NONE', #373, 1000.000000000000000 ) ;
#22441=CARTESIAN_POINT ( 'NONE',  ( 32.81606138205700773, 44.92314894770293421, 79.37823623207320622 ) ) ;
#22445=CYLINDRICAL_SURFACE ( 'NONE', #13355, 2.000000000000001776 ) ;
#22453=CYLINDRICAL_SURFACE ( 'NONE', #23746, 0.5000000000000004441 ) ;
#22506=ORIENTED_EDGE ( 'NONE', *, *, #12974, .F. ) ;
#22530=CARTESIAN_POINT ( 'NONE',  ( 43.23147868389327897, 41.43850569188389699, 79.37823623207322044 ) ) ;
#22534=AXIS2_PLACEMENT_3D ( 'NONE', #7022, #19004, #14871 ) ;
#22537=DIRECTION ( 'NONE',  ( 1.000000000000000000, 0.000000000000000000, 0.000000000000000000 ) ) ;
#22549=DIRECTION ( 'NONE',  ( 0.000000000000000000, 0.000000000000000000, -1.000000000000000000 ) ) ;
#22567=VERTEX_POINT ( 'NONE', #4480 ) ;
#22593=ORIENTED_EDGE ( 'NONE', *, *, #12827, .F. ) ;
#22630=ADVANCED_FACE ( 'NONE', ( #4097 ), #24153, .F. ) ;
#22654=DIRECTION ( 'NONE',  ( 8.758115402030106693E-47, -1.000000000000000000, 3.469446951953613400E-15 ) ) ;
#22679=EDGE_LOOP ( 'NONE', ( #19586, #22593, #77, #21882 ) ) ;
#22689=DIRECTION ( 'NONE',  ( -1.734723475976805122E-16, 0.000000000000000000, -1.000000000000000000 ) ) ;
#22691=CARTESIAN_POINT ( 'NONE',  ( 33.40064408022072939, 40.76768529863396395, 79.57823623207323749 ) ) ;
#22714=TOROIDAL_SURFACE ( 'NONE', #20661, 1.000000000000000000, 1.000000000000000000 ) ;
#22754=CARTESIAN_POINT ( 'NONE',  ( 32.81606138205700773, 44.92314894770294131, 80.37823623207322044 ) ) ;
#22791=DIRECTION ( 'NONE',  ( -1.000000000000000000, 0.000000000000000000, 0.000000000000000000 ) ) ;
#22799=CARTESIAN_POINT ( 'NONE',  ( 31.01606138205699992, 2.823374736507280597E-13, 81.37823623207336254 ) ) ;
#22801=CARTESIAN_POINT ( 'NONE',  ( 45.81606138205700063, 44.92314894770294131, 80.37823623207322044 ) ) ;
#22832=ADVANCED_FACE ( 'NONE', ( #18890 ), #20697, .F. ) ;
#22847=ORIENTED_EDGE ( 'NONE', *, *, #6786, .T. ) ;
#22855=ORIENTED_EDGE ( 'NONE', *, *, #7895, .T. ) ;
#22875=DIRECTION ( 'NONE',  ( 0.000000000000000000, 3.469446951953613400E-15, 1.000000000000000000 ) ) ;
#22912=DIRECTION ( 'NONE',  ( 0.000000000000000000, 0.000000000000000000, -1.000000000000000000 ) ) ;
#22938=ORIENTED_EDGE ( 'NONE', *, *, #14297, .F. ) ;
#22955=DIRECTION ( 'NONE',  ( 0.000000000000000000, -3.469446951953613400E-15, -1.000000000000000000 ) ) ;
#22987=STYLED_ITEM ( 'NONE', ( #25279 ), #25350 ) ;
#23001=PRODUCT_DEFINITION ( 'UNKNOWN', '', #2235, #20856 ) ;
#23123=CARTESIAN_POINT ( 'NONE',  ( 45.61606138205700489, 36.92314894770294131, 81.17823623207323180 ) ) ;
#23125=ORIENTED_EDGE ( 'NONE', *, *, #10543, .T. ) ;
#23172=ADVANCED_FACE ( 'NONE', ( #2362 ), #21702, .T. ) ;
#23227=CARTESIAN_POINT ( 'NONE',  ( 43.23147868389327897, 41.90149715599300606, 79.37823623207322044 ) ) ;
#23302=EDGE_LOOP ( 'NONE', ( #23509, #8082, #5374, #16946 ) ) ;
#23343=ORIENTED_EDGE ( 'NONE', *, *, #251, .F. ) ;
#23348=ORIENTED_EDGE ( 'NONE', *, *, #19495, .F. ) ;
#23349=CARTESIAN_POINT ( 'NONE',  ( 39.81746892067405952, 40.76768529863396395, 79.57823623207323749 ) ) ;
#23353=AXIS2_PLACEMENT_3D ( 'NONE', #16062, #16435, #21870 ) ;
#23365=( NAMED_UNIT ( * ) PLANE_ANGLE_UNIT ( ) SI_UNIT ( $, .RADIAN. ) );
#23415=TOROIDAL_SURFACE ( 'NONE', #16008, 0.9023161253044896801, 0.2000000000000000111 ) ;
#23440=ORIENTED_EDGE ( 'NONE', *, *, #24334, .T. ) ;
#23469=CIRCLE ( 'NONE', #22251, 0.5000000000000004441 ) ;
#23475=CARTESIAN_POINT ( 'NONE',  ( 32.81606138205700773, 34.92314894770294131, 81.17823623207324601 ) ) ;
#23482=VERTEX_POINT ( 'NONE', #3354 ) ;
#23504=VERTEX_POINT ( 'NONE', #5805 ) ;
#23509=ORIENTED_EDGE ( 'NONE', *, *, #14386, .T. ) ;
#23523=LINE ( 'NONE', #3692, #21531 ) ;
#23530=AXIS2_PLACEMENT_3D ( 'NONE', #11861, #2042, #15829 ) ;
#23541=DIRECTION ( 'NONE',  ( 1.734723475976805122E-16, 3.491481338843134933E-15, 1.000000000000000000 ) ) ;
#23551=CARTESIAN_POINT ( 'NONE',  ( 0.000000000000000000, 2.823374736507280597E-13, 81.37823623207336254 ) ) ;
#23553=CIRCLE ( 'NONE', #102, 0.7106531558045068309 ) ;
#23559=TOROIDAL_SURFACE ( 'NONE', #12486, 1.800000000000000044, 0.2000000000000000111 ) ;
#23599=DIRECTION ( 'NONE',  ( -1.734723475976805122E-16, -3.491481338843134933E-15, -1.000000000000000000 ) ) ;
#23720=EDGE_CURVE ( 'NONE', #5143, #10110, #24070, .T. ) ;
#23724=EDGE_CURVE ( 'NONE', #22567, #12430, #492, .T. ) ;
#23746=AXIS2_PLACEMENT_3D ( 'NONE', #20787, #4801, #8819 ) ;
#23754=CARTESIAN_POINT ( 'NONE',  ( 31.81606138205700418, 2.788239579249953820E-13, 80.37823623207336254 ) ) ;
#23755=ORIENTED_EDGE ( 'NONE', *, *, #625, .T. ) ;
#23760=EDGE_LOOP ( 'NONE', ( #19917, #18887, #18271, #2121 ) ) ;
#23769=ORIENTED_EDGE ( 'NONE', *, *, #4566, .F. ) ;
#23772=VERTEX_POINT ( 'NONE', #6315 ) ;
#23787=CARTESIAN_POINT ( 'NONE',  ( 45.81606138205700063, 46.92314894770293421, 79.37823623207319201 ) ) ;
#23789=VERTEX_POINT ( 'NONE', #8246 ) ;
#23824=CYLINDRICAL_SURFACE ( 'NONE', #17622, 1.000000000000000888 ) ;
#23842=CARTESIAN_POINT ( 'NONE',  ( 32.81606138205700773, 34.92314894770293421, 79.37823623207323465 ) ) ;
#23887=DIRECTION ( 'NONE',  ( 0.000000000000000000, 0.000000000000000000, -1.000000000000000000 ) ) ;
#23894=DIRECTION ( 'NONE',  ( 1.000000000000000000, 0.000000000000000000, -0.000000000000000000 ) ) ;
#23895=ORIENTED_EDGE ( 'NONE', *, *, #22162, .F. ) ;
#23907=DIRECTION ( 'NONE',  ( -0.000000000000000000, -3.469446951953613400E-15, -1.000000000000000000 ) ) ;
#23914=EDGE_LOOP ( 'NONE', ( #3036, #2854, #11809, #21326 ) ) ;
#23920=ORIENTED_EDGE ( 'NONE', *, *, #24360, .F. ) ;
#23942=ORIENTED_EDGE ( 'NONE', *, *, #21225, .F. ) ;
#23972=CARTESIAN_POINT ( 'NONE',  ( 45.81606138205700063, 46.92314894770294131, 81.17823623207318917 ) ) ;
#24023=( GEOMETRIC_REPRESENTATION_CONTEXT ( 3 ) GLOBAL_UNCERTAINTY_ASSIGNED_CONTEXT ( ( #3069 ) ) GLOBAL_UNIT_ASSIGNED_CONTEXT ( ( #19515, #23365, #13465 ) ) REPRESENTATION_CONTEXT ( 'NONE', 'WORKASPACE' ) );
#24025=CARTESIAN_POINT ( 'NONE',  ( 45.61606138205700489, 46.92314894770294131, 81.17823623207318917 ) ) ;
#24064=DIRECTION ( 'NONE',  ( 0.000000000000000000, 0.000000000000000000, 1.000000000000000000 ) ) ;
#24070=LINE ( 'NONE', #17920, #18932 ) ;
#24088=FACE_OUTER_BOUND ( 'NONE', #22239, .T. ) ;
#24112=DIRECTION ( 'NONE',  ( -0.000000000000000000, -3.469446951953613400E-15, -1.000000000000000000 ) ) ;
#24116=FACE_OUTER_BOUND ( 'NONE', #15962, .T. ) ;
#24124=FACE_BOUND ( 'NONE', #9908, .T. ) ;
#24150=DIRECTION ( 'NONE',  ( 1.000000000000000000, -0.000000000000000000, 0.000000000000000000 ) ) ;
#24152=AXIS2_PLACEMENT_3D ( 'NONE', #22691, #9061, #4672 ) ;
#24153=PLANE ( 'NONE',  #24641 ) ;
#24230=DIRECTION ( 'NONE',  ( 0.000000000000000000, -1.000000000000000000, 6.938893903907222067E-15 ) ) ;
#24290=CARTESIAN_POINT ( 'NONE',  ( 33.40064408022072939, 41.67000142393845152, 79.57823623207323749 ) ) ;
#24312=ORIENTED_EDGE ( 'NONE', *, *, #6086, .F. ) ;
#24327=CARTESIAN_POINT ( 'NONE',  ( 33.40064408022072939, 40.95934826813394380, 79.52109337493037344 ) ) ;
#24334=EDGE_CURVE ( 'NONE', #12430, #3400, #8250, .T. ) ;
#24335=CARTESIAN_POINT ( 'NONE',  ( 43.81606138205700063, 36.92314894770294131, 81.17823623207323180 ) ) ;
#24342=FACE_OUTER_BOUND ( 'NONE', #7339, .T. ) ;
#24360=EDGE_CURVE ( 'NONE', #1520, #10123, #8350, .T. ) ;
#24380=EDGE_CURVE ( 'NONE', #21638, #9515, #6207, .T. ) ;
#24399=ORIENTED_EDGE ( 'NONE', *, *, #6272, .F. ) ;
#24400=ORIENTED_EDGE ( 'NONE', *, *, #4809, .F. ) ;
#24415=ADVANCED_FACE ( 'NONE', ( #7174 ), #16832, .F. ) ;
#24425=DIRECTION ( 'NONE',  ( 0.000000000000000000, 1.000000000000000000, 0.000000000000000000 ) ) ;
#24455=ORIENTED_EDGE ( 'NONE', *, *, #19038, .T. ) ;
#24470=VERTEX_POINT ( 'NONE', #7038 ) ;
#24481=CARTESIAN_POINT ( 'NONE',  ( 43.23147868389327897, 41.90149715599300606, 79.87823623207322044 ) ) ;
#24522=DIRECTION ( 'NONE',  ( -0.000000000000000000, -3.469446951953613400E-15, -1.000000000000000000 ) ) ;
#24574=VERTEX_POINT ( 'NONE', #17342 ) ;
#24578=DIRECTION ( 'NONE',  ( 0.000000000000000000, 0.000000000000000000, -1.000000000000000000 ) ) ;
#24597=ORIENTED_EDGE ( 'NONE', *, *, #11646, .T. ) ;
#24613=FACE_OUTER_BOUND ( 'NONE', #97, .T. ) ;
#24641=AXIS2_PLACEMENT_3D ( 'NONE', #23787, #21869, #22241 ) ;
#24652=VECTOR ( 'NONE', #22654, 1000.000000000000000 ) ;
#24658=ORIENTED_EDGE ( 'NONE', *, *, #24683, .T. ) ;
#24661=EDGE_CURVE ( 'NONE', #1711, #9404, #4974, .T. ) ;
#24671=DIRECTION ( 'NONE',  ( 0.000000000000000000, 3.469446951953613400E-15, 1.000000000000000000 ) ) ;
#24680=DIRECTION ( 'NONE',  ( -1.000000000000000000, 0.000000000000000000, 0.000000000000000000 ) ) ;
#24683=EDGE_CURVE ( 'NONE', #9125, #23772, #27, .T. ) ;
#24687=DIRECTION ( 'NONE',  ( 0.000000000000000000, -1.000000000000000000, 6.938893903907222067E-15 ) ) ;
#24704=DIRECTION ( 'NONE',  ( 0.000000000000000000, 1.000000000000000000, 0.000000000000000000 ) ) ;
#24718=CARTESIAN_POINT ( 'NONE',  ( 43.81606138205700063, 34.92314894770293421, 79.37823623207323465 ) ) ;
#24727=ADVANCED_FACE ( 'NONE', ( #6248, #24124, #9995 ), #4578, .T. ) ;
#24755=CARTESIAN_POINT ( 'NONE',  ( 33.40064408022072939, 42.57231754924293909, 79.57823623207323749 ) ) ;
#24766=ORIENTED_EDGE ( 'NONE', *, *, #13, .T. ) ;
#24770=FILL_AREA_STYLE ('',( #3777 ) ) ;
#24786=DIRECTION ( 'NONE',  ( 0.000000000000000000, 1.000000000000000000, -3.469446951953613794E-15 ) ) ;
#24802=ORIENTED_EDGE ( 'NONE', *, *, #11481, .T. ) ;
#24843=LINE ( 'NONE', #22799, #5435 ) ;
#24864=CYLINDRICAL_SURFACE ( 'NONE', #24152, 0.2000000000000057288 ) ;
#24874=ORIENTED_EDGE ( 'NONE', *, *, #13272, .T. ) ;
#24898=ORIENTED_EDGE ( 'NONE', *, *, #1385, .F. ) ;
#24955=EDGE_CURVE ( 'NONE', #11694, #5707, #3345, .T. ) ;
#24958=AXIS2_PLACEMENT_3D ( 'NONE', #12996, #16716, #4998 ) ;
#24976=VERTEX_POINT ( 'NONE', #3439 ) ;
#24984=CARTESIAN_POINT ( 'NONE',  ( 36.81465384343994884, 41.90149715599300606, 79.87823623207322044 ) ) ;
#25020=SURFACE_SIDE_STYLE ('',( #21305 ) ) ;
#25060=DIRECTION ( 'NONE',  ( 1.734723475976805122E-16, 3.491481338843134933E-15, 1.000000000000000000 ) ) ;
#25073=DIRECTION ( 'NONE',  ( 0.000000000000000000, 1.000000000000000000, 0.000000000000000000 ) ) ;
#25113=AXIS2_PLACEMENT_3D ( 'NONE', #11555, #13607, #25423 ) ;
#25195=CIRCLE ( 'NONE', #12892, 0.5000000000000004441 ) ;
#25208=AXIS2_PLACEMENT_3D ( 'NONE', #20399, #7000, #8561 ) ;
#25279=PRESENTATION_STYLE_ASSIGNMENT (( #15255 ) ) ;
#25302=DIRECTION ( 'NONE',  ( -0.000000000000000000, 1.000000000000000000, 0.000000000000000000 ) ) ;
#25350=MANIFOLD_SOLID_BREP ( 'Stock-MAS-155-1', #11424 ) ;
#25366=EDGE_CURVE ( 'NONE', #11694, #10306, #13525, .T. ) ;
#25370=ORIENTED_EDGE ( 'NONE', *, *, #2372, .T. ) ;
#25385=TOROIDAL_SURFACE ( 'NONE', #10593, 0.2314957320545545372, 0.5000000000000000000 ) ;
#25397=ORIENTED_EDGE ( 'NONE', *, *, #17615, .T. ) ;
#25400=DIRECTION ( 'NONE',  ( -8.758115402030106693E-47, 1.000000000000000000, -3.469446951953613400E-15 ) ) ;
#25423=DIRECTION ( 'NONE',  ( 1.000000000000000000, 6.938893903907222067E-15, 0.000000000000000000 ) ) ;
#25442=EDGE_CURVE ( 'NONE', #11430, #6274, #19279, .T. ) ;
#25466=ORIENTED_EDGE ( 'NONE', *, *, #5481, .T. ) ;
ENDSEC;
END-ISO-10303-21;
